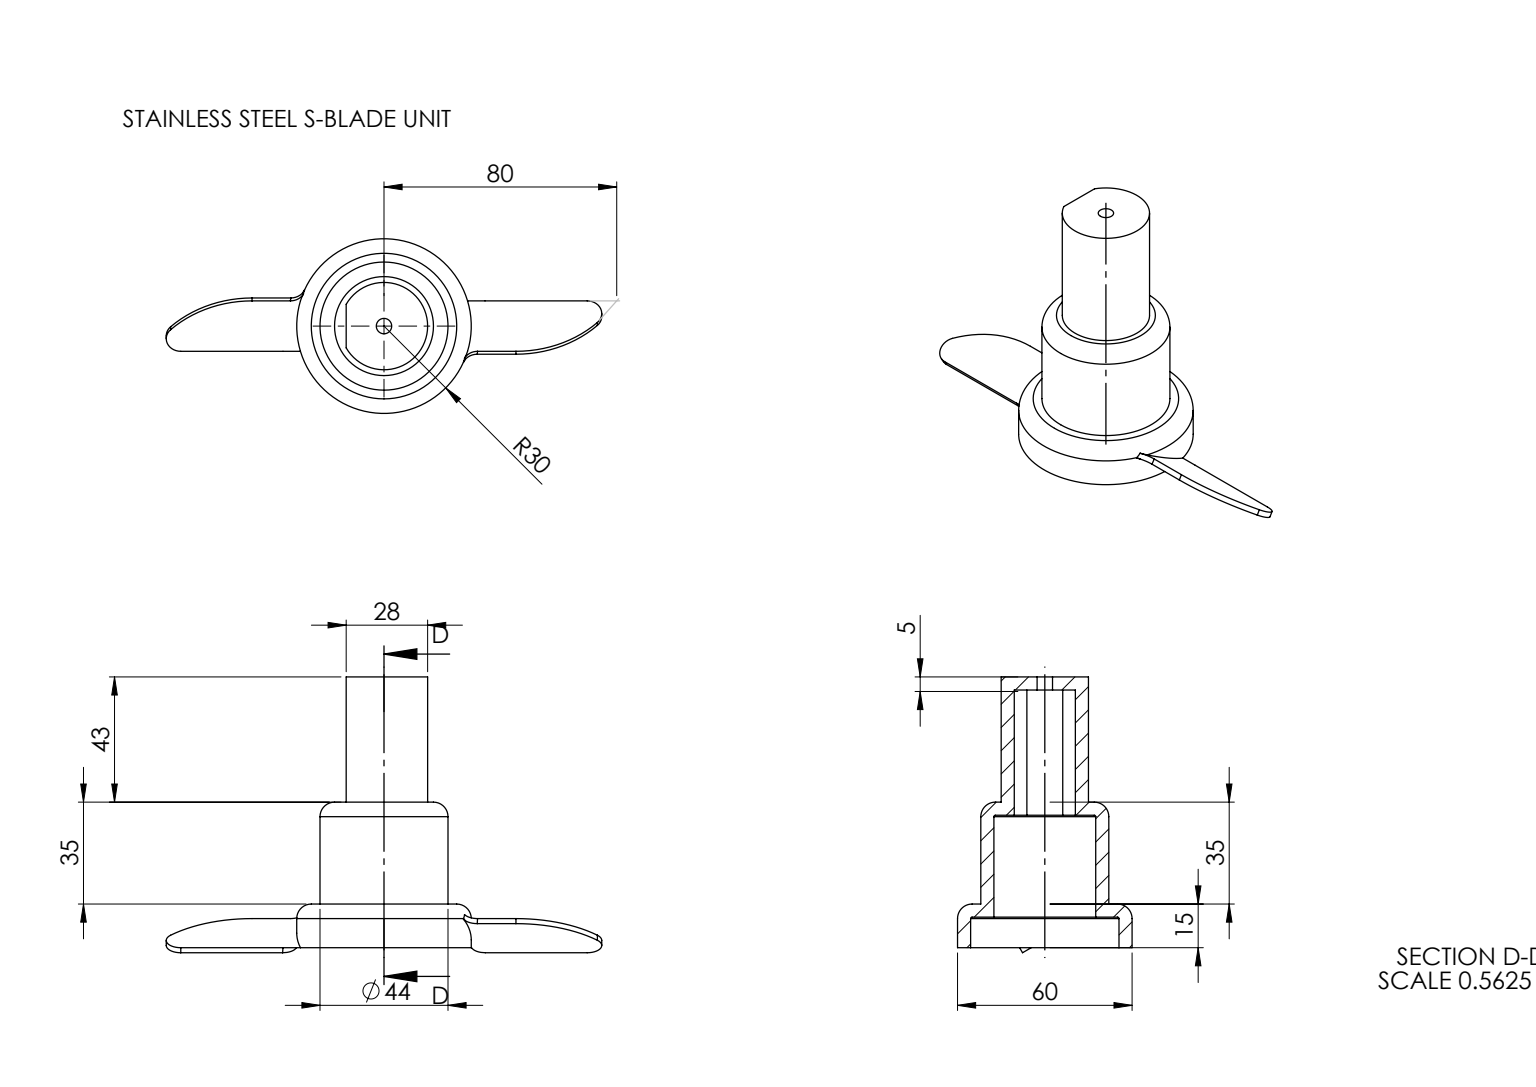
ISO-10303-21;
HEADER;
FILE_DESCRIPTION (('STEP AP214'),
    '1' );
FILE_NAME ('Stainless Steel S-Blade Unit.step',
    '2026-10-08T14:59:03',
    ( '' ),
    ( '' ),
    'SwSTEP 2.0',
    'SolidWorks 2026',
    '' );
FILE_SCHEMA (( 'AUTOMOTIVE_DESIGN' ));
ENDSEC;

DATA;
#5=LINE ( 'NONE', #4817, #10432 ) ;
#8=VERTEX_POINT ( 'NONE', #10428 ) ;
#24=DIRECTION ( 'NONE',  ( 0.000000000000000000, 0.000000000000000000, -1.000000000000000000 ) ) ;
#25=CARTESIAN_POINT ( 'NONE',  ( -30.63265341208206038, 76.40790137508867019, 5.685798939282528330 ) ) ;
#48=EDGE_LOOP ( 'NONE', ( #1031, #6053, #2883, #3031 ) ) ;
#49=CARTESIAN_POINT ( 'NONE',  ( 30.43737458073258040, 77.00000000000001421, -5.702507482421638407 ) ) ;
#59=DIRECTION ( 'NONE',  ( 0.000000000000000000, -0.4999999999999976685, 0.8660254037844399289 ) ) ;
#68=AXIS2_PLACEMENT_3D ( 'NONE', #1472, #532, #4327 ) ;
#76=ORIENTED_EDGE ( 'NONE', *, *, #6927, .T. ) ;
#80=VERTEX_POINT ( 'NONE', #3761 ) ;
#106=DIRECTION ( 'NONE',  ( -0.000000000000000000, -1.000000000000000000, -0.000000000000000000 ) ) ;
#111=ORIENTED_EDGE ( 'NONE', *, *, #6676, .F. ) ;
#114=CARTESIAN_POINT ( 'NONE',  ( 27.33018067101281900, 86.99999999999998579, 12.37179148263487782 ) ) ;
#142=EDGE_LOOP ( 'NONE', ( #5615, #3837, #7263, #6163, #8146, #5499, #6846 ) ) ;
#144=DIRECTION ( 'NONE',  ( -0.000000000000000000, -1.000000000000000000, -0.000000000000000000 ) ) ;
#151=ORIENTED_EDGE ( 'NONE', *, *, #4389, .T. ) ;
#174=CARTESIAN_POINT ( 'NONE',  ( 30.14540500433760783, 76.99999999999997158, -4.927060346216586950 ) ) ;
#181=DIRECTION ( 'NONE',  ( 0.000000000000000000, -0.000000000000000000, 1.000000000000000000 ) ) ;
#182=ORIENTED_EDGE ( 'NONE', *, *, #8491, .F. ) ;
#188=LINE ( 'NONE', #3126, #12048 ) ;
#189=ORIENTED_EDGE ( 'NONE', *, *, #4744, .F. ) ;
#205=ORIENTED_EDGE ( 'NONE', *, *, #4032, .F. ) ;
#207=PRODUCT ( 'Stainless Steel S-Blade Unit', 'Stainless Steel S-Blade Unit', '', ( #412 ) ) ;
#221=TOROIDAL_SURFACE ( 'NONE', #8577, 17.00000000000000000, 5.000000000000000000 ) ;
#224=ADVANCED_FACE ( 'NONE', ( #10291 ), #7552, .F. ) ;
#226=CARTESIAN_POINT ( 'NONE',  ( 31.26438337082144159, 85.29075299833057500, 9.699751388268191832 ) ) ;
#227=CARTESIAN_POINT ( 'NONE',  ( 3.245314017740478073E-16, 170.0000000000000000, -2.649999999999993694 ) ) ;
#228=FACE_OUTER_BOUND ( 'NONE', #12039, .T. ) ;
#230=EDGE_LOOP ( 'NONE', ( #6810, #2498, #7329, #11688 ) ) ;
#247=CYLINDRICAL_SURFACE ( 'NONE', #2591, 40.00000000000000000 ) ;
#248=EDGE_CURVE ( 'NONE', #3797, #2264, #8566, .T. ) ;
#268=ORIENTED_EDGE ( 'NONE', *, *, #4405, .T. ) ;
#281=EDGE_LOOP ( 'NONE', ( #4160, #1583, #966, #3668, #2740 ) ) ;
#283=DIRECTION ( 'NONE',  ( 1.224646799147352714E-16, 0.000000000000000000, -1.000000000000000000 ) ) ;
#293=ADVANCED_FACE ( 'NONE', ( #5930 ), #247, .T. ) ;
#302=VECTOR ( 'NONE', #2224, 1000.000000000000000 ) ;
#311=AXIS2_PLACEMENT_3D ( 'NONE', #7560, #9353, #11370 ) ;
#330=B_SPLINE_CURVE_WITH_KNOTS ( 'NONE', 3,
 ( #6794, #1186, #6609, #4798, #1865, #11603, #5861, #4988, #8525, #7602, #9644, #2863, #10471, #8586, #49, #3865, #174, #7662 ),
 .UNSPECIFIED., .F., .F.,
 ( 4, 2, 2, 2, 2, 2, 2, 2, 4 ),
 ( 2.823925224926892107E-17, 0.0008221565609605404907, 0.001644313121921052792, 0.002466469682881565310, 0.003288626243842077395, 0.004110782804802590347, 0.004932939365763108937, 0.005755095926723627527, 0.006577252487684147851 ),
 .UNSPECIFIED. ) ;
#331=ORIENTED_EDGE ( 'NONE', *, *, #3823, .F. ) ;
#334=VERTEX_POINT ( 'NONE', #4888 ) ;
#373=CARTESIAN_POINT ( 'NONE',  ( 0.000000000000000000, 87.00000000000000000, 0.000000000000000000 ) ) ;
#380=DIRECTION ( 'NONE',  ( 1.000000000000000000, 0.000000000000000000, 0.000000000000000000 ) ) ;
#386=( GEOMETRIC_REPRESENTATION_CONTEXT ( 3 ) GLOBAL_UNCERTAINTY_ASSIGNED_CONTEXT ( ( #5659 ) ) GLOBAL_UNIT_ASSIGNED_CONTEXT ( ( #9241, #4519, #9302 ) ) REPRESENTATION_CONTEXT ( 'NONE', 'WORKASPACE' ) );
#396=CIRCLE ( 'NONE', #7375, 0.5000000000000004441 ) ;
#397=APPLICATION_CONTEXT ( 'automotive_design' ) ;
#408=EDGE_CURVE ( 'NONE', #10035, #8931, #706, .T. ) ;
#412=PRODUCT_CONTEXT ( 'NONE', #6769, 'mechanical' ) ;
#420=TOROIDAL_SURFACE ( 'NONE', #1423, 17.00000000000000000, 5.000000000000000000 ) ;
#422=CARTESIAN_POINT ( 'NONE',  ( 27.33018067101282966, 87.00000000000000000, 12.37179148263486539 ) ) ;
#425=CARTESIAN_POINT ( 'NONE',  ( 1.285879139104720633E-15, 216.0365690573663926, 10.49999999999999822 ) ) ;
#426=EDGE_LOOP ( 'NONE', ( #189, #2218, #6237, #8413 ) ) ;
#427=CIRCLE ( 'NONE', #3428, 30.00000000000000000 ) ;
#429=AXIS2_PLACEMENT_3D ( 'NONE', #2506, #6308, #1510 ) ;
#430=CARTESIAN_POINT ( 'NONE',  ( -30.34950626935404827, 87.16600977219412982, -8.947791397837656646 ) ) ;
#432=DIRECTION ( 'NONE',  ( 0.000000000000000000, 0.000000000000000000, 1.000000000000000000 ) ) ;
#446=LINE ( 'NONE', #10918, #2988 ) ;
#459=DIRECTION ( 'NONE',  ( 0.000000000000000000, 0.000000000000000000, 1.000000000000000000 ) ) ;
#471=CARTESIAN_POINT ( 'NONE',  ( 30.49437064397536901, 76.52118294276679933, -5.489589508502957571 ) ) ;
#497=ORIENTED_EDGE ( 'NONE', *, *, #5720, .F. ) ;
#498=DIRECTION ( 'NONE',  ( -0.000000000000000000, -1.000000000000000000, -0.000000000000000000 ) ) ;
#506=CARTESIAN_POINT ( 'NONE',  ( -29.63582346253862454, 77.00000000000000000, 4.660254037844413944 ) ) ;
#532=DIRECTION ( 'NONE',  ( 0.000000000000000000, 1.000000000000000000, 0.000000000000000000 ) ) ;
#534=CARTESIAN_POINT ( 'NONE',  ( 27.30107202361637775, 86.87046582918780757, 12.43589427268144831 ) ) ;
#535=CARTESIAN_POINT ( 'NONE',  ( 30.15809951803416666, 76.87504465863048608, -4.876683037773544172 ) ) ;
#536=CARTESIAN_POINT ( 'NONE',  ( 0.000000000000000000, 170.0000000000000000, 0.000000000000000000 ) ) ;
#545=PRODUCT_DEFINITION ( 'UNKNOWN', '', #11724, #3142 ) ;
#556=CIRCLE ( 'NONE', #11914, 10.49999999999999822 ) ;
#570=FACE_OUTER_BOUND ( 'NONE', #48, .T. ) ;
#579=DIRECTION ( 'NONE',  ( -1.000000000000000000, 0.000000000000000000, 0.000000000000000000 ) ) ;
#593=DIRECTION ( 'NONE',  ( 0.000000000000000000, 1.000000000000000000, 0.000000000000000000 ) ) ;
#601=CARTESIAN_POINT ( 'NONE',  ( -27.65415084186107109, 87.92311536631548563, -11.47631757750353643 ) ) ;
#614=CARTESIAN_POINT ( 'NONE',  ( 27.65415084186298245, 87.92311536631358138, 11.47631757750026438 ) ) ;
#620=CARTESIAN_POINT ( 'NONE',  ( -27.67899820261485999, 88.38261385519929547, -11.05501148229834030 ) ) ;
#621=ORIENTED_EDGE ( 'NONE', *, *, #3640, .F. ) ;
#625=CIRCLE ( 'NONE', #4207, 5.000000000000000888 ) ;
#626=CARTESIAN_POINT ( 'NONE',  ( 31.12930703771215235, 75.68563247576862807, -7.901403593909491541 ) ) ;
#630=CARTESIAN_POINT ( 'NONE',  ( 69.85388127645428824, 79.49999999999998579, -4.330127018922231841 ) ) ;
#635=CYLINDRICAL_SURFACE ( 'NONE', #1812, 30.00000000000000000 ) ;
#638=EDGE_CURVE ( 'NONE', #7703, #7018, #7140, .T. ) ;
#640=CARTESIAN_POINT ( 'NONE',  ( 27.65180490099799115, 87.90152798314358051, 11.49631016393330540 ) ) ;
#647=ORIENTED_EDGE ( 'NONE', *, *, #8392, .F. ) ;
#657=FILL_AREA_STYLE_COLOUR ( '', #970 ) ;
#661=CARTESIAN_POINT ( 'NONE',  ( -45.35898384862240107, 86.99999999999997158, -8.660254037844424602 ) ) ;
#670=CYLINDRICAL_SURFACE ( 'NONE', #2203, 10.49999999999999822 ) ;
#671=EDGE_CURVE ( 'NONE', #7769, #10587, #7043, .T. ) ;
#674=CYLINDRICAL_SURFACE ( 'NONE', #5648, 15.00000000000000000 ) ;
#676=CARTESIAN_POINT ( 'NONE',  ( -30.00100000000000122, 77.00000000000000000, -8.660254037844445918 ) ) ;
#683=ADVANCED_FACE ( 'NONE', ( #4455, #3529 ), #8312, .T. ) ;
#688=CARTESIAN_POINT ( 'NONE',  ( 34.77127485704751564, 76.44489695195846934, -8.339765143629700006 ) ) ;
#691=DIRECTION ( 'NONE',  ( 0.000000000000000000, -0.8660254037844407060, -0.4999999999999965028 ) ) ;
#696=CYLINDRICAL_SURFACE ( 'NONE', #1896, 17.50000000000000000 ) ;
#703=DIRECTION ( 'NONE',  ( 1.000000000000000000, 0.000000000000000000, 0.000000000000000000 ) ) ;
#706=B_SPLINE_CURVE_WITH_KNOTS ( 'NONE', 3,
 ( #3890, #11502, #7747, #11561 ),
 .UNSPECIFIED., .F., .F.,
 ( 4, 4 ),
 ( 0.000000000000000000, 0.001357209897699670955 ),
 .UNSPECIFIED. ) ;
#718=FACE_OUTER_BOUND ( 'NONE', #11904, .T. ) ;
#721=DIRECTION ( 'NONE',  ( -0.000000000000000000, -1.000000000000000000, -0.000000000000000000 ) ) ;
#722=CIRCLE ( 'NONE', #921, 40.00000000000000000 ) ;
#724=EDGE_LOOP ( 'NONE', ( #7478, #11917, #621, #1398 ) ) ;
#726=B_SPLINE_CURVE_WITH_KNOTS ( 'NONE', 3,
 ( #5759, #4688, #1765, #8421 ),
 .UNSPECIFIED., .F., .F.,
 ( 4, 4 ),
 ( 0.000000000000000000, 0.002001274951694169153 ),
 .UNSPECIFIED. ) ;
#734=CARTESIAN_POINT ( 'NONE',  ( 0.000000000000000000, 127.0000000000000000, 0.000000000000000000 ) ) ;
#742=EDGE_LOOP ( 'NONE', ( #9342, #3526, #10485, #11102, #11036 ) ) ;
#747=ADVANCED_FACE ( 'NONE', ( #10001, #3466 ), #7268, .F. ) ;
#748=DIRECTION ( 'NONE',  ( 0.000000000000000000, 0.000000000000000000, 1.000000000000000000 ) ) ;
#751=ORIENTED_EDGE ( 'NONE', *, *, #7330, .F. ) ;
#754=DIRECTION ( 'NONE',  ( 0.000000000000000000, 1.000000000000000000, 0.000000000000000000 ) ) ;
#757=ORIENTED_EDGE ( 'NONE', *, *, #11505, .F. ) ;
#759=CARTESIAN_POINT ( 'NONE',  ( -34.72842983617974966, 77.03714026276665550, 8.681696978550554888 ) ) ;
#763=MANIFOLD_SOLID_BREP ( 'M5 Clearance Hole1', #5696 ) ;
#771=CARTESIAN_POINT ( 'NONE',  ( 27.52813290908668264, 87.44182241851449078, 11.93450069589769136 ) ) ;
#773=AXIS2_PLACEMENT_3D ( 'NONE', #816, #4609, #12225 ) ;
#781=CARTESIAN_POINT ( 'NONE',  ( -45.35898384862240107, 65.26794919243121740, 24.98076211353317078 ) ) ;
#784=DIRECTION ( 'NONE',  ( 0.000000000000000000, 0.000000000000000000, -1.000000000000000000 ) ) ;
#802=ORIENTED_EDGE ( 'NONE', *, *, #6455, .F. ) ;
#807=CIRCLE ( 'NONE', #9945, 5.000000000000000888 ) ;
#813=AXIS2_PLACEMENT_3D ( 'NONE', #4855, #106, #2049 ) ;
#816=CARTESIAN_POINT ( 'NONE',  ( 0.000000000000000000, 122.5000000000000000, 0.000000000000000000 ) ) ;
#817=DIRECTION ( 'NONE',  ( 0.000000000000000000, 0.000000000000000000, 1.000000000000000000 ) ) ;
#820=CARTESIAN_POINT ( 'NONE',  ( -31.06657576416735012, 76.26187158480907158, 8.234095398640720376 ) ) ;
#852=CARTESIAN_POINT ( 'NONE',  ( -31.33267436902169933, 77.00000000000000000, 7.087639215986555108 ) ) ;
#864=CARTESIAN_POINT ( 'NONE',  ( 0.000000000000000000, 127.0000000000000000, 0.000000000000000000 ) ) ;
#870=CARTESIAN_POINT ( 'NONE',  ( 0.000000000000000000, 77.00000000000000000, 0.000000000000000000 ) ) ;
#897=EDGE_CURVE ( 'NONE', #5507, #7525, #3143, .T. ) ;
#898=ORIENTED_EDGE ( 'NONE', *, *, #2970, .F. ) ;
#913=DIRECTION ( 'NONE',  ( -0.000000000000000000, -1.000000000000000000, -0.000000000000000000 ) ) ;
#921=AXIS2_PLACEMENT_3D ( 'NONE', #781, #3754, #11121 ) ;
#922=UNCERTAINTY_MEASURE_WITH_UNIT (LENGTH_MEASURE( 1.000000000000000082E-05 ), #12072, 'distance_accuracy_value', 'NONE');
#928=CARTESIAN_POINT ( 'NONE',  ( 0.000000000000000000, 170.0000000000000000, 2.649999999999987477 ) ) ;
#929=DIRECTION ( 'NONE',  ( -0.000000000000000000, -1.000000000000000000, -0.000000000000000000 ) ) ;
#931=VERTEX_POINT ( 'NONE', #10744 ) ;
#941=ORIENTED_EDGE ( 'NONE', *, *, #1209, .F. ) ;
#944=DIRECTION ( 'NONE',  ( 0.000000000000000000, 0.000000000000000000, 1.000000000000000000 ) ) ;
#945=VERTEX_POINT ( 'NONE', #2266 ) ;
#948=CYLINDRICAL_SURFACE ( 'NONE', #5812, 25.50000000000000000 ) ;
#949=CARTESIAN_POINT ( 'NONE',  ( 0.000000000000000000, 122.0000000000000000, 0.000000000000000000 ) ) ;
#954=ORIENTED_EDGE ( 'NONE', *, *, #1330, .T. ) ;
#955=FACE_OUTER_BOUND ( 'NONE', #3507, .T. ) ;
#957=DIRECTION ( 'NONE',  ( 1.000000000000000000, 0.000000000000000000, 0.000000000000000000 ) ) ;
#966=ORIENTED_EDGE ( 'NONE', *, *, #9420, .T. ) ;
#970=COLOUR_RGB ( '', 0.72549020, 0.75294118, 0.79215686) ;
#973=EDGE_CURVE ( 'NONE', #8579, #2134, #1216, .T. ) ;
#993=ORIENTED_EDGE ( 'NONE', *, *, #10766, .F. ) ;
#998=ORIENTED_EDGE ( 'NONE', *, *, #9593, .T. ) ;
#1003=CARTESIAN_POINT ( 'NONE',  ( 73.35315233757310693, 81.28571428571424917, -1.237179148263527928 ) ) ;
#1009=ORIENTED_EDGE ( 'NONE', *, *, #2846, .T. ) ;
#1031=ORIENTED_EDGE ( 'NONE', *, *, #1499, .F. ) ;
#1044=DIRECTION ( 'NONE',  ( 0.000000000000000000, 0.000000000000000000, 1.000000000000000000 ) ) ;
#1045=CARTESIAN_POINT ( 'NONE',  ( -30.00100000000000122, 87.00000000000000000, 8.660254037844435260 ) ) ;
#1049=DIRECTION ( 'NONE',  ( 0.000000000000000000, 0.000000000000000000, 1.000000000000000000 ) ) ;
#1058=EDGE_LOOP ( 'NONE', ( #182, #7997, #8845 ) ) ;
#1069=AXIS2_PLACEMENT_3D ( 'NONE', #1304, #9952, #1425 ) ;
#1071=EDGE_CURVE ( 'NONE', #4547, #3216, #10105, .T. ) ;
#1084=DIRECTION ( 'NONE',  ( -1.000000000000000000, 0.000000000000000000, 0.000000000000000000 ) ) ;
#1086=FACE_OUTER_BOUND ( 'NONE', #6691, .T. ) ;
#1091=CIRCLE ( 'NONE', #12038, 2.649999999999993694 ) ;
#1106=AXIS2_PLACEMENT_3D ( 'NONE', #9506, #3916, #8635 ) ;
#1108=CARTESIAN_POINT ( 'NONE',  ( 32.05000697088088657, 85.26794919243110371, 9.660254037844429931 ) ) ;
#1109=CARTESIAN_POINT ( 'NONE',  ( 0.000000000000000000, 170.0000000000000000, 0.000000000000000000 ) ) ;
#1112=VERTEX_POINT ( 'NONE', #10048 ) ;
#1155=DIRECTION ( 'NONE',  ( 0.000000000000000000, 0.000000000000000000, 1.000000000000000000 ) ) ;
#1159=CARTESIAN_POINT ( 'NONE',  ( -31.48070082314331231, 75.91043305631261262, 6.547439342558601716 ) ) ;
#1169=( BOUNDED_CURVE ( )  B_SPLINE_CURVE ( 3, ( #7961, #10837, #3366, #8897 ),
 .UNSPECIFIED., .F., .F. ) 
 B_SPLINE_CURVE_WITH_KNOTS ( ( 4, 4 ),
 ( 1.143370257677567281, 1.145717000886475878 ),
 .UNSPECIFIED. ) 
 CURVE ( )  GEOMETRIC_REPRESENTATION_ITEM ( )  RATIONAL_B_SPLINE_CURVE ( ( 1.000000000000000000, 0.9999995410664119788, 0.9999995410664119788, 1.000000000000000000 ) ) 
 REPRESENTATION_ITEM ( '' )  );
#1177=EDGE_CURVE ( 'NONE', #334, #8, #726, .T. ) ;
#1183=CARTESIAN_POINT ( 'NONE',  ( -69.85388127645425982, 75.26794919243111792, 7.660254037844449471 ) ) ;
#1186=CARTESIAN_POINT ( 'NONE',  ( 34.45294269781049223, 77.00000000000002842, -8.660253777987195534 ) ) ;
#1203=PLANE ( 'NONE',  #10847 ) ;
#1208=CARTESIAN_POINT ( 'NONE',  ( -73.35315233757310693, 79.55366347814538130, 0.2371791482635408899 ) ) ;
#1209=EDGE_CURVE ( 'NONE', #931, #7101, #5, .T. ) ;
#1216=LINE ( 'NONE', #10621, #3070 ) ;
#1230=DIRECTION ( 'NONE',  ( -0.000000000000000000, 1.000000000000000000, -0.000000000000000000 ) ) ;
#1246=CARTESIAN_POINT ( 'NONE',  ( 27.32044479829590244, 86.95653975047672191, 12.39329872843003066 ) ) ;
#1255=ORIENTED_EDGE ( 'NONE', *, *, #4032, .T. ) ;
#1257=CARTESIAN_POINT ( 'NONE',  ( 29.92433840049366012, 87.25972750007186107, 9.110115264091716014 ) ) ;
#1273=VECTOR ( 'NONE', #6369, 1000.000000000000000 ) ;
#1284=VECTOR ( 'NONE', #579, 1000.000000000000000 ) ;
#1285=AXIS2_PLACEMENT_3D ( 'NONE', #870, #2729, #748 ) ;
#1293=CARTESIAN_POINT ( 'NONE',  ( -45.35898384862240107, 67.00000000000008527, 25.98076211353315657 ) ) ;
#1294=CARTESIAN_POINT ( 'NONE',  ( -28.72281323269012532, 77.00000000000000000, 8.660254037844445918 ) ) ;
#1298=VECTOR ( 'NONE', #12093, 1000.000000000000000 ) ;
#1301=EDGE_CURVE ( 'NONE', #5989, #7101, #10232, .T. ) ;
#1304=CARTESIAN_POINT ( 'NONE',  ( 0.000000000000000000, 87.50000000000000000, 0.000000000000000000 ) ) ;
#1307=CARTESIAN_POINT ( 'NONE',  ( 30.00100000000000122, 77.00000000000000000, 8.660254037844445918 ) ) ;
#1309=VECTOR ( 'NONE', #6876, 1000.000000000000000 ) ;
#1318=DIRECTION ( 'NONE',  ( 0.000000000000000000, 0.000000000000000000, 1.000000000000000000 ) ) ;
#1330=EDGE_CURVE ( 'NONE', #7513, #6899, #8632, .T. ) ;
#1364=CARTESIAN_POINT ( 'NONE',  ( 34.73110591274434000, 77.00000000000000000, -8.660254037844445918 ) ) ;
#1368=CARTESIAN_POINT ( 'NONE',  ( -29.32777202433393526, 87.43477800909944619, -9.413311639618301641 ) ) ;
#1386=CARTESIAN_POINT ( 'NONE',  ( 28.72281323269012532, 87.00000000000000000, 8.660254037844435260 ) ) ;
#1393=ORIENTED_EDGE ( 'NONE', *, *, #5864, .F. ) ;
#1398=ORIENTED_EDGE ( 'NONE', *, *, #4341, .T. ) ;
#1399=CARTESIAN_POINT ( 'NONE',  ( 45.35898384862240107, 5.499999999999840128, 9.526279441628638267 ) ) ;
#1409=AXIS2_PLACEMENT_3D ( 'NONE', #11572, #5209, #459 ) ;
#1413=CARTESIAN_POINT ( 'NONE',  ( 30.00100000000000122, 87.00000000000000000, -8.660254037844435260 ) ) ;
#1414=CIRCLE ( 'NONE', #5603, 22.00000000000000355 ) ;
#1415=CARTESIAN_POINT ( 'NONE',  ( 33.79339916392899568, 75.30908861350523864, -7.588998470350058589 ) ) ;
#1423=AXIS2_PLACEMENT_3D ( 'NONE', #949, #4556, #8530 ) ;
#1425=DIRECTION ( 'NONE',  ( 0.000000000000000000, 0.000000000000000000, 1.000000000000000000 ) ) ;
#1426=ORIENTED_EDGE ( 'NONE', *, *, #1301, .F. ) ;
#1436=ORIENTED_EDGE ( 'NONE', *, *, #4623, .T. ) ;
#1439=LINE ( 'NONE', #11859, #12313 ) ;
#1443=CARTESIAN_POINT ( 'NONE',  ( 0.000000000000000000, 127.0000000000000000, 0.000000000000000000 ) ) ;
#1445=ORIENTED_EDGE ( 'NONE', *, *, #1071, .F. ) ;
#1448=CARTESIAN_POINT ( 'NONE',  ( -30.55518048406710818, 80.37544454677752981, -1.186187415305626436 ) ) ;
#1449=DIRECTION ( 'NONE',  ( 0.000000000000000000, 0.000000000000000000, -1.000000000000000000 ) ) ;
#1450=ORIENTED_EDGE ( 'NONE', *, *, #3823, .T. ) ;
#1453=ORIENTED_EDGE ( 'NONE', *, *, #9437, .F. ) ;
#1454=EDGE_CURVE ( 'NONE', #7484, #7525, #4811, .T. ) ;
#1472=CARTESIAN_POINT ( 'NONE',  ( 0.000000000000000000, 77.00000000000000000, 0.000000000000000000 ) ) ;
#1482=CARTESIAN_POINT ( 'NONE',  ( 69.85388127645425982, 75.26794919243111792, -7.660254037844449471 ) ) ;
#1486=CARTESIAN_POINT ( 'NONE',  ( 31.88521078284829713, 87.00000000000001421, 14.43375672974067569 ) ) ;
#1499=EDGE_CURVE ( 'NONE', #9385, #11869, #4012, .T. ) ;
#1510=DIRECTION ( 'NONE',  ( 0.000000000000000000, -0.4999999999999976130, -0.8660254037844400399 ) ) ;
#1513=CARTESIAN_POINT ( 'NONE',  ( 28.47250777504872588, 87.47929846073044757, 9.490423323819145551 ) ) ;
#1538=CARTESIAN_POINT ( 'NONE',  ( -31.92904760676809062, 76.99999999999998579, 7.658217335466646070 ) ) ;
#1548=ORIENTED_EDGE ( 'NONE', *, *, #4290, .T. ) ;
#1554=DIRECTION ( 'NONE',  ( 0.000000000000000000, 1.000000000000000000, 0.000000000000000000 ) ) ;
#1557=CARTESIAN_POINT ( 'NONE',  ( -28.14852131675075242, 87.98519278820045031, -10.36665800225805967 ) ) ;
#1558=ADVANCED_FACE ( 'NONE', ( #11038 ), #221, .T. ) ;
#1559=ORIENTED_EDGE ( 'NONE', *, *, #6927, .F. ) ;
#1569=VERTEX_POINT ( 'NONE', #3245 ) ;
#1583=ORIENTED_EDGE ( 'NONE', *, *, #4955, .T. ) ;
#1593=DIRECTION ( 'NONE',  ( 0.000000000000000000, 1.000000000000000000, 0.000000000000000000 ) ) ;
#1600=CARTESIAN_POINT ( 'NONE',  ( -27.56105762898379652, 86.58728811733517716, -11.86287969473305814 ) ) ;
#1607=ADVANCED_FACE ( 'NONE', ( #4426 ), #8219, .F. ) ;
#1612=AXIS2_PLACEMENT_3D ( 'NONE', #9562, #7823, #5032 ) ;
#1614=DIRECTION ( 'NONE',  ( 0.000000000000000000, 0.8660254037844405950, 0.4999999999999965028 ) ) ;
#1617=CARTESIAN_POINT ( 'NONE',  ( 27.96741528345890870, 86.27927944434865992, 11.41192941739706335 ) ) ;
#1626=CARTESIAN_POINT ( 'NONE',  ( 2.081899558550500280E-15, 122.0000000000000000, -17.00000000000000000 ) ) ;
#1630=AXIS2_PLACEMENT_3D ( 'NONE', #2809, #11358, #8265 ) ;
#1637=DIRECTION ( 'NONE',  ( 1.224646799147357151E-16, 0.000000000000000000, -1.000000000000000000 ) ) ;
#1642=DIRECTION ( 'NONE',  ( -0.000000000000000000, -1.000000000000000000, -0.000000000000000000 ) ) ;
#1643=( BOUNDED_CURVE ( )  B_SPLINE_CURVE ( 3, ( #3135, #10732, #5077, #8852 ),
 .UNSPECIFIED., .F., .F. ) 
 B_SPLINE_CURVE_WITH_KNOTS ( ( 4, 4 ),
 ( 1.666086958916892291, 1.694832046014206117 ),
 .UNSPECIFIED. ) 
 CURVE ( )  GEOMETRIC_REPRESENTATION_ITEM ( )  RATIONAL_B_SPLINE_CURVE ( ( 1.000000000000000000, 0.9999311445159493328, 0.9999311445159493328, 1.000000000000000000 ) ) 
 REPRESENTATION_ITEM ( '' )  );
#1653=ORIENTED_EDGE ( 'NONE', *, *, #8115, .F. ) ;
#1657=EDGE_CURVE ( 'NONE', #3216, #11487, #625, .T. ) ;
#1659=CARTESIAN_POINT ( 'NONE',  ( -34.45294269781049223, 77.00000000000002842, 8.660253777987195534 ) ) ;
#1661=CARTESIAN_POINT ( 'NONE',  ( -28.82113438504157799, 85.77482169909444565, -9.367611059671812512 ) ) ;
#1663=CARTESIAN_POINT ( 'NONE',  ( 1.285879139104720633E-15, 165.5000000000000000, 10.49999999999999822 ) ) ;
#1667=ADVANCED_FACE ( 'NONE', ( #3848 ), #10176, .T. ) ;
#1671=STYLED_ITEM ( 'NONE', ( #11321 ), #763 ) ;
#1675=CARTESIAN_POINT ( 'NONE',  ( -69.85388127645428824, 75.26794919243114634, 7.660254037844465458 ) ) ;
#1677=DIRECTION ( 'NONE',  ( -0.000000000000000000, -1.000000000000000000, -0.000000000000000000 ) ) ;
#1679=EDGE_LOOP ( 'NONE', ( #3569, #5275 ) ) ;
#1685=CARTESIAN_POINT ( 'NONE',  ( 31.18707241436460365, 75.10640101998821194, -7.566984156997462740 ) ) ;
#1689=DIRECTION ( 'NONE',  ( 0.000000000000000000, 1.000000000000000000, 0.000000000000000000 ) ) ;
#1690=CARTESIAN_POINT ( 'NONE',  ( -34.84179752789421514, 75.25738092153642356, 7.654152443798540872 ) ) ;
#1705=PLANE ( 'NONE',  #7184 ) ;
#1718=SURFACE_STYLE_USAGE ( .BOTH. , #10116 ) ;
#1719=AXIS2_PLACEMENT_3D ( 'NONE', #8085, #1554, #2298 ) ;
#1720=CIRCLE ( 'NONE', #8675, 5.000000000000000000 ) ;
#1723=CARTESIAN_POINT ( 'NONE',  ( -30.55702146375036676, 77.00000000000001421, 5.949569453687718834 ) ) ;
#1732=AXIS2_PLACEMENT_3D ( 'NONE', #4755, #7623, #8611 ) ;
#1736=DIRECTION ( 'NONE',  ( 0.000000000000000000, 0.000000000000000000, 1.000000000000000000 ) ) ;
#1739=FACE_BOUND ( 'NONE', #6832, .T. ) ;
#1745=CARTESIAN_POINT ( 'NONE',  ( 31.06657576416735012, 76.26187158480907158, -8.234095398640720376 ) ) ;
#1746=CARTESIAN_POINT ( 'NONE',  ( 30.43816488677641630, 83.71535165408627677, 2.971076217724753832 ) ) ;
#1756=CIRCLE ( 'NONE', #10100, 10.49999999999999822 ) ;
#1760=EDGE_CURVE ( 'NONE', #5507, #8953, #9981, .T. ) ;
#1761=ORIENTED_EDGE ( 'NONE', *, *, #7465, .F. ) ;
#1765=CARTESIAN_POINT ( 'NONE',  ( 32.14616437604218646, 85.84037417286381810, 9.329764321300741514 ) ) ;
#1778=CARTESIAN_POINT ( 'NONE',  ( -30.83210227225915290, 77.00000000000000000, 6.426308247889123137 ) ) ;
#1783=LINE ( 'NONE', #9186, #2910 ) ;
#1793=VERTEX_POINT ( 'NONE', #8756 ) ;
#1795=DIRECTION ( 'NONE',  ( 0.000000000000000000, 0.000000000000000000, 1.000000000000000000 ) ) ;
#1799=B_SPLINE_CURVE_WITH_KNOTS ( 'NONE', 3,
 ( #9122, #535, #10819, #471, #4398, #9817, #7147, #7089, #3412, #11832, #10944, #1415, #12015, #8193 ),
 .UNSPECIFIED., .F., .F.,
 ( 4, 2, 2, 2, 2, 2, 4 ),
 ( 0.001978049138782353184, 0.002761379211137155940, 0.003544709283491958261, 0.004328039355846760583, 0.005111369428201563772, 0.006678029572911168416, 0.008244689717620771324 ),
 .UNSPECIFIED. ) ;
#1812=AXIS2_PLACEMENT_3D ( 'NONE', #4187, #3447, #1449 ) ;
#1822=EDGE_CURVE ( 'NONE', #9024, #5307, #10195, .T. ) ;
#1825=ORIENTED_EDGE ( 'NONE', *, *, #7480, .T. ) ;
#1827=CYLINDRICAL_SURFACE ( 'NONE', #311, 10.49999999999999822 ) ;
#1828=ORIENTED_EDGE ( 'NONE', *, *, #2846, .F. ) ;
#1831=AXIS2_PLACEMENT_3D ( 'NONE', #10884, #3158, #9815 ) ;
#1834=VERTEX_POINT ( 'NONE', #6029 ) ;
#1836=EDGE_CURVE ( 'NONE', #10799, #1569, #9879, .T. ) ;
#1837=CARTESIAN_POINT ( 'NONE',  ( 0.000000000000000000, 92.00000000000000000, -25.50000000000000000 ) ) ;
#1840=DIRECTION ( 'NONE',  ( -1.000000000000000000, 0.000000000000000000, 0.000000000000000000 ) ) ;
#1845=EDGE_CURVE ( 'NONE', #1793, #9034, #5023, .T. ) ;
#1854=AXIS2_PLACEMENT_3D ( 'NONE', #4718, #10633, #4846 ) ;
#1858=ORIENTED_EDGE ( 'NONE', *, *, #1499, .T. ) ;
#1865=CARTESIAN_POINT ( 'NONE',  ( 33.37417589188917333, 76.99999999999998579, -8.451338748825380165 ) ) ;
#1872=VECTOR ( 'NONE', #9243, 1000.000000000000000 ) ;
#1873=ORIENTED_EDGE ( 'NONE', *, *, #897, .F. ) ;
#1879=FACE_BOUND ( 'NONE', #2862, .T. ) ;
#1881=ORIENTED_EDGE ( 'NONE', *, *, #6930, .T. ) ;
#1882=VECTOR ( 'NONE', #957, 1000.000000000000000 ) ;
#1885=EDGE_LOOP ( 'NONE', ( #8424, #7096, #8090, #5651 ) ) ;
#1886=EDGE_CURVE ( 'NONE', #2508, #11122, #427, .T. ) ;
#1896=AXIS2_PLACEMENT_3D ( 'NONE', #10342, #2625, #9283 ) ;
#1897=EDGE_LOOP ( 'NONE', ( #10651, #7896, #3999, #10787, #1426, #9113, #4225, #8537, #9822 ) ) ;
#1900=SURFACE_STYLE_USAGE ( .BOTH. , #9368 ) ;
#1903=DIRECTION ( 'NONE',  ( 0.000000000000000000, 0.000000000000000000, 1.000000000000000000 ) ) ;
#1904=DIRECTION ( 'NONE',  ( 0.000000000000000000, 1.000000000000000000, 0.000000000000000000 ) ) ;
#1918=CARTESIAN_POINT ( 'NONE',  ( -69.85388127645428824, 77.76794919243110371, 3.330127018922237614 ) ) ;
#1932=AXIS2_PLACEMENT_3D ( 'NONE', #5152, #8871, #3211 ) ;
#1939=DIRECTION ( 'NONE',  ( 0.000000000000000000, -0.8660254037844407060, 0.4999999999999965028 ) ) ;
#1947=EDGE_LOOP ( 'NONE', ( #4493, #4209, #2967, #5069 ) ) ;
#1957=CIRCLE ( 'NONE', #2153, 15.00000000000000000 ) ;
#1985=STYLED_ITEM ( 'NONE', ( #11194 ), #4372 ) ;
#2011=DIRECTION ( 'NONE',  ( 0.000000000000000000, 0.000000000000000000, 1.000000000000000000 ) ) ;
#2019=EDGE_CURVE ( 'NONE', #5470, #8579, #11159, .T. ) ;
#2033=CARTESIAN_POINT ( 'NONE',  ( -30.25776724459628753, 76.75431408359612817, 5.085794527760020500 ) ) ;
#2040=DIRECTION ( 'NONE',  ( 0.000000000000000000, 0.4999999999999962808, 0.8660254037844407060 ) ) ;
#2041=( BOUNDED_SURFACE ( )  B_SPLINE_SURFACE ( 3, 2, ( 
 ( #422, #4344, #6287 ),
 ( #8948, #3423, #2353 ),
 ( #614, #3294, #7097 ),
 ( #9131, #3232, #6042 ) ),
 .UNSPECIFIED., .F., .F., .F. ) 
 B_SPLINE_SURFACE_WITH_KNOTS ( ( 4, 4 ),
 ( 3, 3 ),
 ( 0.08252307147638787699, 0.08572545668793386808 ),
 ( 0.000000000000000000, 1.000000000000000000 ),
 .UNSPECIFIED. ) 
 GEOMETRIC_REPRESENTATION_ITEM ( )  RATIONAL_B_SPLINE_SURFACE ( (
 ( 1.000000000000000000, 0.8237544710479146604, 1.000000000000000000),
 ( 1.000000000000000000, 0.8337078205039558654, 1.000000000000000000),
 ( 1.000000000000000000, 0.8426243553970736988, 1.000000000000000000),
 ( 1.000000000000000000, 0.8507194741069452615, 1.000000000000000000) ) ) 
 REPRESENTATION_ITEM ( '' )  SURFACE ( )  );
#2049=DIRECTION ( 'NONE',  ( 0.000000000000000000, 0.000000000000000000, -1.000000000000000000 ) ) ;
#2051=ORIENTED_EDGE ( 'NONE', *, *, #4623, .F. ) ;
#2061=CARTESIAN_POINT ( 'NONE',  ( 0.000000000000000000, 87.00000000000000000, 0.000000000000000000 ) ) ;
#2075=VECTOR ( 'NONE', #3237, 1000.000000000000000 ) ;
#2076=FACE_OUTER_BOUND ( 'NONE', #10289, .T. ) ;
#2085=EDGE_CURVE ( 'NONE', #4062, #4534, #5791, .T. ) ;
#2089=EDGE_LOOP ( 'NONE', ( #9140, #4210, #268, #10094 ) ) ;
#2095=VECTOR ( 'NONE', #1614, 1000.000000000000000 ) ;
#2105=DIRECTION ( 'NONE',  ( 0.000000000000000000, -0.8660254037844402619, -0.4999999999999975575 ) ) ;
#2114=CARTESIAN_POINT ( 'NONE',  ( -34.73110591274434000, 77.00000000000000000, 8.660254037844445918 ) ) ;
#2119=VERTEX_POINT ( 'NONE', #5837 ) ;
#2121=DIRECTION ( 'NONE',  ( -1.000000000000000000, 0.000000000000000000, 0.000000000000000000 ) ) ;
#2134=VERTEX_POINT ( 'NONE', #6706 ) ;
#2147=FACE_OUTER_BOUND ( 'NONE', #2962, .T. ) ;
#2153=AXIS2_PLACEMENT_3D ( 'NONE', #9084, #6545, #5305 ) ;
#2157=ORIENTED_EDGE ( 'NONE', *, *, #2279, .F. ) ;
#2173=ORIENTED_EDGE ( 'NONE', *, *, #3226, .F. ) ;
#2183=EDGE_CURVE ( 'NONE', #7236, #5974, #11966, .T. ) ;
#2186=CARTESIAN_POINT ( 'NONE',  ( 0.000000000000000000, 92.00000000000000000, 0.000000000000000000 ) ) ;
#2201=ORIENTED_EDGE ( 'NONE', *, *, #3226, .T. ) ;
#2203=AXIS2_PLACEMENT_3D ( 'NONE', #3595, #5413, #2656 ) ;
#2208=ORIENTED_EDGE ( 'NONE', *, *, #2759, .T. ) ;
#2218=ORIENTED_EDGE ( 'NONE', *, *, #5864, .T. ) ;
#2222=DIRECTION ( 'NONE',  ( -1.000000000000000000, 0.000000000000000000, 0.000000000000000000 ) ) ;
#2223=CARTESIAN_POINT ( 'NONE',  ( -27.33018067101282256, 87.00000000000000000, -12.37179148263487605 ) ) ;
#2224=DIRECTION ( 'NONE',  ( -1.000000000000000000, 0.000000000000000000, 0.000000000000000000 ) ) ;
#2229=CARTESIAN_POINT ( 'NONE',  ( 0.000000000000000000, 165.5000000000000000, 0.000000000000000000 ) ) ;
#2232=FACE_OUTER_BOUND ( 'NONE', #9916, .T. ) ;
#2233=EDGE_CURVE ( 'NONE', #7634, #1834, #7698, .T. ) ;
#2235=ORIENTED_EDGE ( 'NONE', *, *, #10451, .T. ) ;
#2264=VERTEX_POINT ( 'NONE', #7878 ) ;
#2266=CARTESIAN_POINT ( 'NONE',  ( 34.73110591274434000, 77.00000000000000000, -8.660254037844445918 ) ) ;
#2277=CIRCLE ( 'NONE', #1285, 25.50000000000000000 ) ;
#2279=EDGE_CURVE ( 'NONE', #3932, #7967, #5569, .T. ) ;
#2281=DIRECTION ( 'NONE',  ( 0.000000000000000000, 0.8660254037844405950, -0.4999999999999965028 ) ) ;
#2290=DIRECTION ( 'NONE',  ( 0.000000000000000000, 0.000000000000000000, -1.000000000000000000 ) ) ;
#2294=ORIENTED_EDGE ( 'NONE', *, *, #4258, .T. ) ;
#2297=CARTESIAN_POINT ( 'NONE',  ( 34.84121487603211875, 75.26794919243111792, -7.660254037844449471 ) ) ;
#2298=DIRECTION ( 'NONE',  ( 0.000000000000000000, 0.000000000000000000, 1.000000000000000000 ) ) ;
#2304=TOROIDAL_SURFACE ( 'NONE', #2708, 24.99999999999999645, 0.5000000000000004441 ) ;
#2309=CARTESIAN_POINT ( 'NONE',  ( 32.15778161310143446, 87.00000000000000000, 8.660254037844435260 ) ) ;
#2320=CARTESIAN_POINT ( 'NONE',  ( 3.061616997868382648E-15, 87.00000000000000000, -24.99999999999999645 ) ) ;
#2327=CARTESIAN_POINT ( 'NONE',  ( 30.00100000000000122, 75.26794919243111792, 7.660254037844449471 ) ) ;
#2330=DIRECTION ( 'NONE',  ( 0.000000000000000000, 0.8660254037844407060, -0.4999999999999965583 ) ) ;
#2339=CARTESIAN_POINT ( 'NONE',  ( -29.42287733398164207, 85.62135522733750292, -10.27237124600374685 ) ) ;
#2344=AXIS2_PLACEMENT_3D ( 'NONE', #4238, #3309, #1318 ) ;
#2353=CARTESIAN_POINT ( 'NONE',  ( 32.12519652190606223, 85.41823950547951938, 9.573483885149325801 ) ) ;
#2366=CARTESIAN_POINT ( 'NONE',  ( 29.32777202433393526, 87.43477800909943198, 9.413311639618298088 ) ) ;
#2374=DIRECTION ( 'NONE',  ( 0.000000000000000000, 0.000000000000000000, 1.000000000000000000 ) ) ;
#2399=CYLINDRICAL_SURFACE ( 'NONE', #5552, 5.000000000000000000 ) ;
#2401=CARTESIAN_POINT ( 'NONE',  ( -27.52813290908667909, 87.44182241851447657, -11.93450069589770202 ) ) ;
#2412=ADVANCED_FACE ( 'NONE', ( #7499 ), #1705, .T. ) ;
#2416=EDGE_LOOP ( 'NONE', ( #6778, #2617, #12291, #4175 ) ) ;
#2425=CARTESIAN_POINT ( 'NONE',  ( -31.23312648697675797, 87.04033007153444146, -8.730107770814976575 ) ) ;
#2429=DIRECTION ( 'NONE',  ( -1.000000000000000000, 0.000000000000000000, 0.000000000000000000 ) ) ;
#2431=EDGE_LOOP ( 'NONE', ( #7696, #7036, #9329, #5583 ) ) ;
#2453=ORIENTED_EDGE ( 'NONE', *, *, #6299, .T. ) ;
#2467=CARTESIAN_POINT ( 'NONE',  ( 0.000000000000000000, 170.0000000000000000, 0.000000000000000000 ) ) ;
#2469=LINE ( 'NONE', #10816, #7444 ) ;
#2483=CARTESIAN_POINT ( 'NONE',  ( -8.500000000000000000, 165.5000000000000000, -6.164414002968973350 ) ) ;
#2487=ORIENTED_EDGE ( 'NONE', *, *, #10672, .T. ) ;
#2492=CARTESIAN_POINT ( 'NONE',  ( 2.143131898507868248E-15, 87.50000000000000000, 17.50000000000000000 ) ) ;
#2498=ORIENTED_EDGE ( 'NONE', *, *, #6710, .T. ) ;
#2506=CARTESIAN_POINT ( 'NONE',  ( 69.85388127645428824, 77.76794919243110371, -3.330127018922237614 ) ) ;
#2508=VERTEX_POINT ( 'NONE', #10293 ) ;
#2518=( BOUNDED_CURVE ( )  B_SPLINE_CURVE ( 3, ( #2803, #3521, #7324, #11123 ),
 .UNSPECIFIED., .F., .F. ) 
 B_SPLINE_CURVE_WITH_KNOTS ( ( 4, 4 ),
 ( 4.419546208656112363, 5.005231752113266985 ),
 .UNSPECIFIED. ) 
 CURVE ( )  GEOMETRIC_REPRESENTATION_ITEM ( )  RATIONAL_B_SPLINE_CURVE ( ( 1.000000000000000000, 0.9716180718375584391, 0.9716180718375584391, 1.000000000000000000 ) ) 
 REPRESENTATION_ITEM ( '' )  );
#2519=EDGE_LOOP ( 'NONE', ( #3043, #898, #6208, #10217 ) ) ;
#2523=DIRECTION ( 'NONE',  ( -0.000000000000000000, 1.000000000000000000, -0.000000000000000000 ) ) ;
#2529=EDGE_LOOP ( 'NONE', ( #10134, #941, #10729, #6130, #6110, #9810, #9335, #11430, #3942 ) ) ;
#2531=CARTESIAN_POINT ( 'NONE',  ( -32.05000697088088657, 85.26794919243110371, -9.660254037844429931 ) ) ;
#2534=CARTESIAN_POINT ( 'NONE',  ( -27.96269517408193295, 86.23182228119658532, -11.42938571145656113 ) ) ;
#2558=DIRECTION ( 'NONE',  ( 1.000000000000000000, -0.000000000000000000, 1.224646799147353207E-16 ) ) ;
#2559=CARTESIAN_POINT ( 'NONE',  ( -34.77127485704751564, 76.44489695195846934, 8.339765143629700006 ) ) ;
#2568=CARTESIAN_POINT ( 'NONE',  ( 27.67899820261485999, 88.38261385519929547, 11.05501148229834030 ) ) ;
#2591=AXIS2_PLACEMENT_3D ( 'NONE', #12353, #11489, #59 ) ;
#2593=CARTESIAN_POINT ( 'NONE',  ( 69.85388127645425982, 77.00000000000000000, -8.660254037844445918 ) ) ;
#2610=EDGE_LOOP ( 'NONE', ( #10047, #6944, #9511, #1873 ) ) ;
#2616=CARTESIAN_POINT ( 'NONE',  ( 1.285879139104720633E-15, 122.5000000000000000, 10.49999999999999822 ) ) ;
#2617=ORIENTED_EDGE ( 'NONE', *, *, #2746, .T. ) ;
#2621=AXIS2_PLACEMENT_3D ( 'NONE', #6498, #2684, #12234 ) ;
#2625=DIRECTION ( 'NONE',  ( -0.000000000000000000, -1.000000000000000000, -0.000000000000000000 ) ) ;
#2627=DIRECTION ( 'NONE',  ( 0.000000000000000000, 1.000000000000000000, 0.000000000000000000 ) ) ;
#2632=ADVANCED_FACE ( 'NONE', ( #955, #1879 ), #7676, .F. ) ;
#2640=FACE_OUTER_BOUND ( 'NONE', #2416, .T. ) ;
#2645=CIRCLE ( 'NONE', #6630, 17.00000000000000000 ) ;
#2649=CARTESIAN_POINT ( 'NONE',  ( -32.15133482848810331, 77.00000000000000000, 7.827692000169491848 ) ) ;
#2655=AXIS2_PLACEMENT_3D ( 'NONE', #11585, #10574, #2040 ) ;
#2656=DIRECTION ( 'NONE',  ( 0.000000000000000000, 0.000000000000000000, -1.000000000000000000 ) ) ;
#2662=VECTOR ( 'NONE', #7873, 1000.000000000000000 ) ;
#2666=ORIENTED_EDGE ( 'NONE', *, *, #8899, .T. ) ;
#2669=EDGE_LOOP ( 'NONE', ( #6979, #8099, #1828, #6259 ) ) ;
#2674=CARTESIAN_POINT ( 'NONE',  ( 0.000000000000000000, 165.5000000000000000, 0.000000000000000000 ) ) ;
#2683=AXIS2_PLACEMENT_3D ( 'NONE', #10168, #1642, #5449 ) ;
#2684=DIRECTION ( 'NONE',  ( 0.000000000000000000, -0.4999999999999965028, -0.8660254037844407060 ) ) ;
#2708=AXIS2_PLACEMENT_3D ( 'NONE', #5329, #9170, #11185 ) ;
#2724=ORIENTED_EDGE ( 'NONE', *, *, #7617, .F. ) ;
#2729=DIRECTION ( 'NONE',  ( 0.000000000000000000, 1.000000000000000000, 0.000000000000000000 ) ) ;
#2740=ORIENTED_EDGE ( 'NONE', *, *, #9346, .T. ) ;
#2742=DIRECTION ( 'NONE',  ( -0.000000000000000000, 0.4999999999999965028, 0.8660254037844407060 ) ) ;
#2746=EDGE_CURVE ( 'NONE', #5955, #11632, #8787, .T. ) ;
#2751=VECTOR ( 'NONE', #12258, 1000.000000000000000 ) ;
#2759=EDGE_CURVE ( 'NONE', #2264, #334, #11255, .T. ) ;
#2764=ORIENTED_EDGE ( 'NONE', *, *, #1822, .F. ) ;
#2765=( NAMED_UNIT ( * ) PLANE_ANGLE_UNIT ( ) SI_UNIT ( $, .RADIAN. ) );
#2766=EDGE_CURVE ( 'NONE', #1112, #11439, #1439, .T. ) ;
#2771=AXIS2_PLACEMENT_3D ( 'NONE', #10562, #4768, #24 ) ;
#2775=B_SPLINE_CURVE_WITH_KNOTS ( 'NONE', 3,
 ( #1617, #6538, #6352, #10325 ),
 .UNSPECIFIED., .F., .F.,
 ( 4, 4 ),
 ( 0.000000000000000000, 0.001357209897699809299 ),
 .UNSPECIFIED. ) ;
#2787=EDGE_CURVE ( 'NONE', #10587, #5507, #5939, .T. ) ;
#2790=PRODUCT_DEFINITION_SHAPE ( 'NONE', 'NONE',  #545 ) ;
#2800=FACE_OUTER_BOUND ( 'NONE', #2529, .T. ) ;
#2803=CARTESIAN_POINT ( 'NONE',  ( -28.72281323269012887, 87.00000000000000000, -8.660254037844435260 ) ) ;
#2806=EDGE_CURVE ( 'NONE', #2508, #945, #10970, .T. ) ;
#2809=CARTESIAN_POINT ( 'NONE',  ( -31.88521078284829713, 86.99999999999998579, -14.43375672974068991 ) ) ;
#2830=ADVANCED_FACE ( 'NONE', ( #6928 ), #10724, .F. ) ;
#2833=ORIENTED_EDGE ( 'NONE', *, *, #1657, .F. ) ;
#2841=( BOUNDED_CURVE ( )  B_SPLINE_CURVE ( 3, ( #8964, #1746, #3616, #3799 ),
 .UNSPECIFIED., .F., .F. ) 
 B_SPLINE_CURVE_WITH_KNOTS ( ( 4, 4 ),
 ( 4.419546208656112363, 5.005231752113266985 ),
 .UNSPECIFIED. ) 
 CURVE ( )  GEOMETRIC_REPRESENTATION_ITEM ( )  RATIONAL_B_SPLINE_CURVE ( ( 1.000000000000000000, 0.9716180718375584391, 0.9716180718375584391, 1.000000000000000000 ) ) 
 REPRESENTATION_ITEM ( '' )  );
#2844=EDGE_CURVE ( 'NONE', #4062, #7080, #11713, .T. ) ;
#2846=EDGE_CURVE ( 'NONE', #7525, #7634, #1957, .T. ) ;
#2853=EDGE_LOOP ( 'NONE', ( #3610, #6946, #1825, #10648 ) ) ;
#2856=CARTESIAN_POINT ( 'NONE',  ( 0.000000000000000000, 122.0000000000000000, 17.00000000000000000 ) ) ;
#2862=EDGE_LOOP ( 'NONE', ( #2918, #6840 ) ) ;
#2863=CARTESIAN_POINT ( 'NONE',  ( 30.98881549816775660, 77.00000000000001421, -6.657310619789788220 ) ) ;
#2883=ORIENTED_EDGE ( 'NONE', *, *, #10339, .T. ) ;
#2888=EDGE_CURVE ( 'NONE', #8670, #4839, #1756, .T. ) ;
#2903=CARTESIAN_POINT ( 'NONE',  ( -32.32195836398363298, 75.59155356138302295, 7.099754829268524858 ) ) ;
#2910=VECTOR ( 'NONE', #4647, 1000.000000000000000 ) ;
#2915=ADVANCED_FACE ( 'NONE', ( #10085 ), #11031, .T. ) ;
#2918=ORIENTED_EDGE ( 'NONE', *, *, #4353, .T. ) ;
#2927=DIRECTION ( 'NONE',  ( 0.000000000000000000, 1.000000000000000000, 0.000000000000000000 ) ) ;
#2948=ORIENTED_EDGE ( 'NONE', *, *, #4601, .T. ) ;
#2958=VECTOR ( 'NONE', #3371, 1000.000000000000000 ) ;
#2962=EDGE_LOOP ( 'NONE', ( #76, #10415 ) ) ;
#2963=DIRECTION ( 'NONE',  ( 0.000000000000000000, 0.000000000000000000, 1.000000000000000000 ) ) ;
#2967=ORIENTED_EDGE ( 'NONE', *, *, #10354, .T. ) ;
#2968=ORIENTED_EDGE ( 'NONE', *, *, #2806, .F. ) ;
#2970=EDGE_CURVE ( 'NONE', #3368, #6910, #556, .T. ) ;
#2974=EDGE_CURVE ( 'NONE', #8555, #7080, #10511, .T. ) ;
#2975=EDGE_CURVE ( 'NONE', #11714, #7098, #7526, .T. ) ;
#2980=CARTESIAN_POINT ( 'NONE',  ( -32.14616437604218646, 85.84037417286381810, -9.329764321300741514 ) ) ;
#2988=VECTOR ( 'NONE', #703, 1000.000000000000000 ) ;
#3025=CARTESIAN_POINT ( 'NONE',  ( 0.000000000000000000, 165.5000000000000000, 2.649999999999993694 ) ) ;
#3028=LINE ( 'NONE', #9682, #8873 ) ;
#3030=ORIENTED_EDGE ( 'NONE', *, *, #408, .F. ) ;
#3031=ORIENTED_EDGE ( 'NONE', *, *, #4877, .F. ) ;
#3033=ORIENTED_EDGE ( 'NONE', *, *, #6455, .T. ) ;
#3035=CARTESIAN_POINT ( 'NONE',  ( 0.000000000000000000, 92.00000000000000000, 24.99999999999999645 ) ) ;
#3036=DIRECTION ( 'NONE',  ( 0.000000000000000000, 1.000000000000000000, 0.000000000000000000 ) ) ;
#3042=AXIS2_PLACEMENT_3D ( 'NONE', #7697, #913, #6827 ) ;
#3043=ORIENTED_EDGE ( 'NONE', *, *, #6726, .F. ) ;
#3048=TOROIDAL_SURFACE ( 'NONE', #11820, 24.99999999999999645, 0.5000000000000004441 ) ;
#3070=VECTOR ( 'NONE', #5085, 1000.000000000000000 ) ;
#3073=EDGE_CURVE ( 'NONE', #10304, #11439, #7914, .T. ) ;
#3074=FACE_OUTER_BOUND ( 'NONE', #426, .T. ) ;
#3090=TOROIDAL_SURFACE ( 'NONE', #7477, 17.00000000000000000, 0.5000000000000004441 ) ;
#3093=VECTOR ( 'NONE', #6841, 1000.000000000000000 ) ;
#3106=CYLINDRICAL_SURFACE ( 'NONE', #813, 30.00000000000000000 ) ;
#3110=CARTESIAN_POINT ( 'NONE',  ( -73.35315233757310693, 81.28571428571424917, 1.237179148263527928 ) ) ;
#3126=CARTESIAN_POINT ( 'NONE',  ( 0.000000000000000000, 127.0000000000000000, -17.50000000000000000 ) ) ;
#3133=DIRECTION ( 'NONE',  ( 0.000000000000000000, -0.8660254037844401509, 0.4999999999999974465 ) ) ;
#3134=CARTESIAN_POINT ( 'NONE',  ( -27.30107202361637775, 86.87046582918780757, -12.43589427268144831 ) ) ;
#3135=CARTESIAN_POINT ( 'NONE',  ( -34.84121487603211875, 75.26794919243111792, 7.660254037844449471 ) ) ;
#3142=PRODUCT_DEFINITION_CONTEXT ( 'detailed design', #397, 'design' ) ;
#3143=LINE ( 'NONE', #8684, #2662 ) ;
#3158=DIRECTION ( 'NONE',  ( 0.000000000000000000, 1.000000000000000000, 0.000000000000000000 ) ) ;
#3177=CARTESIAN_POINT ( 'NONE',  ( -29.14112381217239900, 87.50172632198250255, -9.529269519012833811 ) ) ;
#3180=CIRCLE ( 'NONE', #9739, 0.5000000000000004441 ) ;
#3186=CARTESIAN_POINT ( 'NONE',  ( 27.88763417807735578, 88.17431669512683357, 10.69423021798056084 ) ) ;
#3195=DIRECTION ( 'NONE',  ( -0.000000000000000000, -1.000000000000000000, -0.000000000000000000 ) ) ;
#3201=VECTOR ( 'NONE', #721, 1000.000000000000000 ) ;
#3211=DIRECTION ( 'NONE',  ( 0.000000000000000000, 0.000000000000000000, 1.000000000000000000 ) ) ;
#3214=CIRCLE ( 'NONE', #7400, 25.50000000000000000 ) ;
#3216=VERTEX_POINT ( 'NONE', #1183 ) ;
#3220=AXIS2_PLACEMENT_3D ( 'NONE', #536, #7211, #8260 ) ;
#3226=EDGE_CURVE ( 'NONE', #80, #10035, #11498, .T. ) ;
#3227=ADVANCED_FACE ( 'NONE', ( #10940 ), #2399, .T. ) ;
#3231=VERTEX_POINT ( 'NONE', #3110 ) ;
#3232=CARTESIAN_POINT ( 'NONE',  ( 29.05832229253450549, 87.09380371750550864, 8.606096436291641893 ) ) ;
#3237=DIRECTION ( 'NONE',  ( -0.000000000000000000, -1.000000000000000000, -0.000000000000000000 ) ) ;
#3238=CARTESIAN_POINT ( 'NONE',  ( -28.78580657183879765, 87.64875042622799128, -9.783922737503317535 ) ) ;
#3245=CARTESIAN_POINT ( 'NONE',  ( 3.245314017740474622E-16, 170.0000000000000000, -2.649999999999987477 ) ) ;
#3258=CARTESIAN_POINT ( 'NONE',  ( -30.00100000000000122, 85.26794919243110371, 9.660254037844429931 ) ) ;
#3273=VECTOR ( 'NONE', #10824, 1000.000000000000000 ) ;
#3281=LINE ( 'NONE', #1413, #302 ) ;
#3294=CARTESIAN_POINT ( 'NONE',  ( 29.00531465893917371, 86.42397445337759621, 8.992822542244239159 ) ) ;
#3309=DIRECTION ( 'NONE',  ( 0.000000000000000000, 1.000000000000000000, 0.000000000000000000 ) ) ;
#3327=ORIENTED_EDGE ( 'NONE', *, *, #11690, .T. ) ;
#3334=EDGE_CURVE ( 'NONE', #4135, #10304, #3586, .T. ) ;
#3335=DIRECTION ( 'NONE',  ( 0.000000000000000000, 1.000000000000000000, 0.000000000000000000 ) ) ;
#3349=AXIS2_PLACEMENT_3D ( 'NONE', #10588, #2927, #10524 ) ;
#3366=CARTESIAN_POINT ( 'NONE',  ( 27.32050286291078933, 86.95679894682506017, 12.39317045950328300 ) ) ;
#3367=CARTESIAN_POINT ( 'NONE',  ( -28.61611180472258553, 87.72948999988449259, -9.923767781257849308 ) ) ;
#3368=VERTEX_POINT ( 'NONE', #7573 ) ;
#3371=DIRECTION ( 'NONE',  ( -0.000000000000000000, -1.000000000000000000, -0.000000000000000000 ) ) ;
#3394=ORIENTED_EDGE ( 'NONE', *, *, #1836, .T. ) ;
#3405=UNCERTAINTY_MEASURE_WITH_UNIT (LENGTH_MEASURE( 1.000000000000000082E-05 ), #8494, 'distance_accuracy_value', 'NONE');
#3412=CARTESIAN_POINT ( 'NONE',  ( 31.68100721119781937, 75.82462385531685811, -6.696065238440062295 ) ) ;
#3423=CARTESIAN_POINT ( 'NONE',  ( 28.82113438502227609, 85.77482169911409926, 9.367611059682538155 ) ) ;
#3428=AXIS2_PLACEMENT_3D ( 'NONE', #8939, #7829, #5039 ) ;
#3438=DIRECTION ( 'NONE',  ( 0.000000000000000000, 0.000000000000000000, 1.000000000000000000 ) ) ;
#3447=DIRECTION ( 'NONE',  ( -0.000000000000000000, -1.000000000000000000, -0.000000000000000000 ) ) ;
#3461=EDGE_LOOP ( 'NONE', ( #10813, #8441, #1881 ) ) ;
#3466=FACE_OUTER_BOUND ( 'NONE', #1897, .T. ) ;
#3485=ADVANCED_FACE ( 'NONE', ( #2147, #7695 ), #8622, .T. ) ;
#3494=DIRECTION ( 'NONE',  ( 0.000000000000000000, -0.000000000000000000, 1.000000000000000000 ) ) ;
#3503=DIRECTION ( 'NONE',  ( -0.000000000000000000, -1.000000000000000000, -0.000000000000000000 ) ) ;
#3507=EDGE_LOOP ( 'NONE', ( #7921, #2157 ) ) ;
#3515=EDGE_CURVE ( 'NONE', #9969, #9385, #8064, .T. ) ;
#3520=ORIENTED_EDGE ( 'NONE', *, *, #2888, .T. ) ;
#3521=CARTESIAN_POINT ( 'NONE',  ( -30.43816488677641630, 83.71535165408627677, -2.971076217724753832 ) ) ;
#3526=ORIENTED_EDGE ( 'NONE', *, *, #248, .F. ) ;
#3529=FACE_OUTER_BOUND ( 'NONE', #10150, .T. ) ;
#3530=CARTESIAN_POINT ( 'NONE',  ( -30.50145854323920602, 85.38003226577613702, -9.854387615546507107 ) ) ;
#3532=DIRECTION ( 'NONE',  ( 0.000000000000000000, -0.8660254037844402619, 0.4999999999999975575 ) ) ;
#3543=DIRECTION ( 'NONE',  ( 0.000000000000000000, 0.000000000000000000, -1.000000000000000000 ) ) ;
#3544=DIRECTION ( 'NONE',  ( 0.000000000000000000, 1.000000000000000000, 0.000000000000000000 ) ) ;
#3553=CARTESIAN_POINT ( 'NONE',  ( 34.84179752789421514, 75.25738092153642356, -7.654152443798540872 ) ) ;
#3564=FACE_BOUND ( 'NONE', #7875, .T. ) ;
#3565=ORIENTED_EDGE ( 'NONE', *, *, #4744, .T. ) ;
#3569=ORIENTED_EDGE ( 'NONE', *, *, #2183, .T. ) ;
#3586=LINE ( 'NONE', #1837, #2751 ) ;
#3594=AXIS2_PLACEMENT_3D ( 'NONE', #6723, #4158, #2290 ) ;
#3595=CARTESIAN_POINT ( 'NONE',  ( 0.000000000000000000, 216.0365690573663926, 0.000000000000000000 ) ) ;
#3596=AXIS2_PLACEMENT_3D ( 'NONE', #5590, #1904, #4835 ) ;
#3609=EDGE_CURVE ( 'NONE', #4534, #4062, #5705, .T. ) ;
#3610=ORIENTED_EDGE ( 'NONE', *, *, #11582, .F. ) ;
#3613=ORIENTED_EDGE ( 'NONE', *, *, #1071, .T. ) ;
#3616=CARTESIAN_POINT ( 'NONE',  ( 30.43816488677641985, 80.28464834591375165, -2.971076217724743618 ) ) ;
#3640=EDGE_CURVE ( 'NONE', #11487, #5761, #722, .T. ) ;
#3651=ADVANCED_FACE ( 'NONE', ( #12125 ), #1827, .F. ) ;
#3652=CARTESIAN_POINT ( 'NONE',  ( -27.54203853141981995, 86.50063778822037364, -11.90690952824024329 ) ) ;
#3668=ORIENTED_EDGE ( 'NONE', *, *, #9330, .F. ) ;
#3676=CARTESIAN_POINT ( 'NONE',  ( 0.000000000000000000, 87.50000000000000000, 0.000000000000000000 ) ) ;
#3677=DIRECTION ( 'NONE',  ( 0.000000000000000000, 0.000000000000000000, 1.000000000000000000 ) ) ;
#3688=CIRCLE ( 'NONE', #1106, 10.49999999999999822 ) ;
#3736=DIRECTION ( 'NONE',  ( -0.000000000000000000, 0.8660254037844402619, -0.4999999999999975575 ) ) ;
#3737=EDGE_LOOP ( 'NONE', ( #9152, #11526 ) ) ;
#3741=DIRECTION ( 'NONE',  ( -0.000000000000000000, -1.000000000000000000, -0.000000000000000000 ) ) ;
#3754=DIRECTION ( 'NONE',  ( 0.000000000000000000, -0.8660254037844402619, -0.4999999999999975575 ) ) ;
#3761=CARTESIAN_POINT ( 'NONE',  ( -32.05000697088088657, 85.26794919243110371, -9.660254037844429931 ) ) ;
#3769=DIRECTION ( 'NONE',  ( 0.000000000000000000, 1.000000000000000000, 0.000000000000000000 ) ) ;
#3770=CIRCLE ( 'NONE', #6956, 2.649999999999987477 ) ;
#3783=CARTESIAN_POINT ( 'NONE',  ( 27.96741528345890870, 86.27927944434865992, 11.41192941739706335 ) ) ;
#3797=VERTEX_POINT ( 'NONE', #10607 ) ;
#3799=CARTESIAN_POINT ( 'NONE',  ( 28.72281323269012532, 77.00000000000000000, -8.660254037844445918 ) ) ;
#3800=ORIENTED_EDGE ( 'NONE', *, *, #973, .T. ) ;
#3813=AXIS2_PLACEMENT_3D ( 'NONE', #12043, #6493, #691 ) ;
#3817=DIRECTION ( 'NONE',  ( 0.000000000000000000, 1.000000000000000000, 0.000000000000000000 ) ) ;
#3823=EDGE_CURVE ( 'NONE', #8953, #7769, #5760, .T. ) ;
#3834=SURFACE_STYLE_FILL_AREA ( #11446 ) ;
#3837=ORIENTED_EDGE ( 'NONE', *, *, #7456, .T. ) ;
#3840=CARTESIAN_POINT ( 'NONE',  ( -31.68100721119781937, 75.82462385531685811, 6.696065238440062295 ) ) ;
#3848=FACE_OUTER_BOUND ( 'NONE', #11983, .T. ) ;
#3865=CARTESIAN_POINT ( 'NONE',  ( 30.23169114332096896, 76.99999999999998579, -5.192055827170280580 ) ) ;
#3867=ORIENTED_EDGE ( 'NONE', *, *, #6315, .T. ) ;
#3890=CARTESIAN_POINT ( 'NONE',  ( -27.96741528345882344, 86.27927944434871677, -11.41192941739715927 ) ) ;
#3916=DIRECTION ( 'NONE',  ( 0.000000000000000000, 1.000000000000000000, 0.000000000000000000 ) ) ;
#3932=VERTEX_POINT ( 'NONE', #11734 ) ;
#3942=ORIENTED_EDGE ( 'NONE', *, *, #5719, .T. ) ;
#3963=CARTESIAN_POINT ( 'NONE',  ( -32.78711330112231792, 75.47285661897714704, 7.305343964218459440 ) ) ;
#3970=CARTESIAN_POINT ( 'NONE',  ( 28.48065962374913695, 85.97961707684491728, 10.89289897176416666 ) ) ;
#3989=CARTESIAN_POINT ( 'NONE',  ( 27.96269517408201821, 86.23182228119654269, 11.42938571145646875 ) ) ;
#3990=EDGE_LOOP ( 'NONE', ( #10978, #1858, #1559, #8988 ) ) ;
#3991=ADVANCED_FACE ( 'NONE', ( #10216 ), #7038, .T. ) ;
#3999=ORIENTED_EDGE ( 'NONE', *, *, #4145, .T. ) ;
#4003=CARTESIAN_POINT ( 'NONE',  ( -13.00000000000000178, 170.0000000000000000, -7.483314773547880883 ) ) ;
#4008=PLANE ( 'NONE',  #1732 ) ;
#4012=CIRCLE ( 'NONE', #4403, 5.000000000000000888 ) ;
#4016=EDGE_CURVE ( 'NONE', #4117, #8618, #1720, .T. ) ;
#4027=CARTESIAN_POINT ( 'NONE',  ( -30.49437064397536901, 76.52118294276679933, 5.489589508502957571 ) ) ;
#4029=EDGE_LOOP ( 'NONE', ( #8804, #4229, #9177, #1653, #10623, #205, #5758, #3565 ) ) ;
#4032=EDGE_CURVE ( 'NONE', #5307, #10772, #11206, .T. ) ;
#4033=FACE_OUTER_BOUND ( 'NONE', #2610, .T. ) ;
#4051=ORIENTED_EDGE ( 'NONE', *, *, #3073, .F. ) ;
#4062=VERTEX_POINT ( 'NONE', #5801 ) ;
#4073=DIRECTION ( 'NONE',  ( 0.000000000000000000, 0.000000000000000000, 1.000000000000000000 ) ) ;
#4116=( BOUNDED_CURVE ( )  B_SPLINE_CURVE ( 3, ( #2297, #9769, #7899, #1364 ),
 .UNSPECIFIED., .F., .F. ) 
 B_SPLINE_CURVE_WITH_KNOTS ( ( 4, 4 ),
 ( 1.666086958916892291, 1.694832046014206117 ),
 .UNSPECIFIED. ) 
 CURVE ( )  GEOMETRIC_REPRESENTATION_ITEM ( )  RATIONAL_B_SPLINE_CURVE ( ( 1.000000000000000000, 0.9999311445159493328, 0.9999311445159493328, 1.000000000000000000 ) ) 
 REPRESENTATION_ITEM ( '' )  );
#4117=VERTEX_POINT ( 'NONE', #1003 ) ;
#4121=CARTESIAN_POINT ( 'NONE',  ( 29.71888078761409346, 87.31388704012290702, 9.203922339174773981 ) ) ;
#4124=DIRECTION ( 'NONE',  ( -0.000000000000000000, -1.000000000000000000, -0.000000000000000000 ) ) ;
#4130=ORIENTED_EDGE ( 'NONE', *, *, #2970, .T. ) ;
#4135=VERTEX_POINT ( 'NONE', #7725 ) ;
#4145=EDGE_CURVE ( 'NONE', #945, #931, #330, .T. ) ;
#4157=ORIENTED_EDGE ( 'NONE', *, *, #5520, .T. ) ;
#4158=DIRECTION ( 'NONE',  ( -0.000000000000000000, -1.000000000000000000, -0.000000000000000000 ) ) ;
#4160=ORIENTED_EDGE ( 'NONE', *, *, #7644, .T. ) ;
#4171=CARTESIAN_POINT ( 'NONE',  ( -29.71888078761410767, 87.31388704012290702, -9.203922339174775757 ) ) ;
#4175=ORIENTED_EDGE ( 'NONE', *, *, #4419, .F. ) ;
#4187=CARTESIAN_POINT ( 'NONE',  ( 0.000000000000000000, 92.00000000000000000, 0.000000000000000000 ) ) ;
#4207=AXIS2_PLACEMENT_3D ( 'NONE', #1918, #2105, #9570 ) ;
#4209=ORIENTED_EDGE ( 'NONE', *, *, #3515, .T. ) ;
#4210=ORIENTED_EDGE ( 'NONE', *, *, #2844, .T. ) ;
#4220=CARTESIAN_POINT ( 'NONE',  ( 3.367778697655220913E-15, 92.00000000000000000, -24.99999999999999645 ) ) ;
#4225=ORIENTED_EDGE ( 'NONE', *, *, #7597, .T. ) ;
#4226=DIRECTION ( 'NONE',  ( 0.000000000000000000, 0.000000000000000000, 1.000000000000000000 ) ) ;
#4229=ORIENTED_EDGE ( 'NONE', *, *, #6676, .T. ) ;
#4231=LINE ( 'NONE', #10778, #2075 ) ;
#4234=CIRCLE ( 'NONE', #11217, 5.000000000000000000 ) ;
#4236=ADVANCED_FACE ( 'NONE', ( #2232 ), #9893, .T. ) ;
#4238=CARTESIAN_POINT ( 'NONE',  ( 0.000000000000000000, 170.0000000000000000, 0.000000000000000000 ) ) ;
#4249=CARTESIAN_POINT ( 'NONE',  ( 28.12254474901590484, 87.93978760833334718, 10.28801392380147206 ) ) ;
#4258=EDGE_CURVE ( 'NONE', #10229, #945, #4116, .T. ) ;
#4276=CIRCLE ( 'NONE', #8046, 2.649999999999993694 ) ;
#4277=CARTESIAN_POINT ( 'NONE',  ( -27.67899820261485999, 88.38261385519929547, -11.05501148229834030 ) ) ;
#4290=EDGE_CURVE ( 'NONE', #7703, #10799, #4276, .T. ) ;
#4299=EDGE_LOOP ( 'NONE', ( #7130, #2764, #4727, #2173, #1393 ) ) ;
#4300=DIRECTION ( 'NONE',  ( 1.000000000000000000, 0.000000000000000000, 0.000000000000000000 ) ) ;
#4303=TOROIDAL_SURFACE ( 'NONE', #6700, 24.99999999999999645, 5.000000000000000000 ) ;
#4304=DIRECTION ( 'NONE',  ( 1.224646799147353454E-16, 0.000000000000000000, -1.000000000000000000 ) ) ;
#4307=CARTESIAN_POINT ( 'NONE',  ( 0.000000000000000000, 127.0000000000000000, 0.000000000000000000 ) ) ;
#4327=DIRECTION ( 'NONE',  ( 0.000000000000000000, -0.000000000000000000, 1.000000000000000000 ) ) ;
#4330=CARTESIAN_POINT ( 'NONE',  ( 30.55518048406710818, 80.37544454677752981, 1.186187415305626436 ) ) ;
#4341=EDGE_CURVE ( 'NONE', #11487, #3231, #11282, .T. ) ;
#4344=CARTESIAN_POINT ( 'NONE',  ( 28.52887280570638495, 85.15789473684209554, 9.723794007404251261 ) ) ;
#4346=DIRECTION ( 'NONE',  ( 0.000000000000000000, 0.000000000000000000, 1.000000000000000000 ) ) ;
#4353=EDGE_CURVE ( 'NONE', #7098, #11714, #11656, .T. ) ;
#4358=FACE_BOUND ( 'NONE', #9792, .T. ) ;
#4361=ORIENTED_EDGE ( 'NONE', *, *, #6169, .T. ) ;
#4364=VERTEX_POINT ( 'NONE', #9198 ) ;
#4368=ORIENTED_EDGE ( 'NONE', *, *, #408, .T. ) ;
#4372=ADVANCED_BREP_SHAPE_REPRESENTATION ( '', ( #763, #1612 ), #10102 ) ;
#4383=CARTESIAN_POINT ( 'NONE',  ( -27.30107202361637775, 86.87046582918780757, -12.43589427268144831 ) ) ;
#4389=EDGE_CURVE ( 'NONE', #945, #8618, #4597, .T. ) ;
#4394=CARTESIAN_POINT ( 'NONE',  ( -30.98881549816775660, 77.00000000000001421, 6.657310619789788220 ) ) ;
#4396=CARTESIAN_POINT ( 'NONE',  ( -32.21610632499845650, 86.34645847305816346, -9.037576414350890985 ) ) ;
#4398=CARTESIAN_POINT ( 'NONE',  ( 30.63265341208206038, 76.40790137508867019, -5.685798939282528330 ) ) ;
#4403=AXIS2_PLACEMENT_3D ( 'NONE', #9970, #2558, #4304 ) ;
#4405=EDGE_CURVE ( 'NONE', #7080, #8555, #10646, .T. ) ;
#4408=CARTESIAN_POINT ( 'NONE',  ( 28.72281323269012532, 87.00000000000000000, 8.660254037844435260 ) ) ;
#4419=EDGE_CURVE ( 'NONE', #6910, #4839, #11147, .T. ) ;
#4423=CARTESIAN_POINT ( 'NONE',  ( 30.03968734988933420, 77.39454232463201322, -4.824121477407818048 ) ) ;
#4424=DIRECTION ( 'NONE',  ( 0.000000000000000000, 1.000000000000000000, 0.000000000000000000 ) ) ;
#4426=FACE_OUTER_BOUND ( 'NONE', #9300, .T. ) ;
#4435=VECTOR ( 'NONE', #817, 1000.000000000000000 ) ;
#4453=FILL_AREA_STYLE ('',( #657 ) ) ;
#4455=FACE_BOUND ( 'NONE', #9008, .T. ) ;
#4456=CARTESIAN_POINT ( 'NONE',  ( -69.85388127645428824, 17.99999999999971223, -31.17691453623957543 ) ) ;
#4457=CARTESIAN_POINT ( 'NONE',  ( 0.000000000000000000, 127.0000000000000000, -15.00000000000000000 ) ) ;
#4460=CARTESIAN_POINT ( 'NONE',  ( 0.000000000000000000, 122.5000000000000000, -10.49999999999999822 ) ) ;
#4473=CARTESIAN_POINT ( 'NONE',  ( 0.000000000000000000, 216.0365690573663926, 0.000000000000000000 ) ) ;
#4475=LINE ( 'NONE', #1675, #10465 ) ;
#4477=LINE ( 'NONE', #7531, #6653 ) ;
#4481=ORIENTED_EDGE ( 'NONE', *, *, #2746, .F. ) ;
#4493=ORIENTED_EDGE ( 'NONE', *, *, #5646, .F. ) ;
#4494=ADVANCED_FACE ( 'NONE', ( #6289 ), #9133, .T. ) ;
#4499=DIRECTION ( 'NONE',  ( 0.000000000000000000, 1.000000000000000000, 0.000000000000000000 ) ) ;
#4505=AXIS2_PLACEMENT_3D ( 'NONE', #1293, #5104, #6216 ) ;
#4509=ORIENTED_EDGE ( 'NONE', *, *, #7456, .F. ) ;
#4511=CARTESIAN_POINT ( 'NONE',  ( 0.000000000000000000, 122.0000000000000000, 0.000000000000000000 ) ) ;
#4515=DIRECTION ( 'NONE',  ( 0.000000000000000000, 0.000000000000000000, 1.000000000000000000 ) ) ;
#4519=( NAMED_UNIT ( * ) PLANE_ANGLE_UNIT ( ) SI_UNIT ( $, .RADIAN. ) );
#4522=AXIS2_PLACEMENT_3D ( 'NONE', #8348, #4499, #8289 ) ;
#4528=DIRECTION ( 'NONE',  ( 0.000000000000000000, 1.000000000000000000, 0.000000000000000000 ) ) ;
#4532=CARTESIAN_POINT ( 'NONE',  ( -30.07733313487553772, 77.00000000000709122, 4.660254037819535178 ) ) ;
#4534=VERTEX_POINT ( 'NONE', #7650 ) ;
#4538=PLANE ( 'NONE',  #6265 ) ;
#4545=CARTESIAN_POINT ( 'NONE',  ( 34.72842983617974966, 77.03714026276665550, -8.681696978550554888 ) ) ;
#4547=VERTEX_POINT ( 'NONE', #6654 ) ;
#4556=DIRECTION ( 'NONE',  ( 0.000000000000000000, 1.000000000000000000, 0.000000000000000000 ) ) ;
#4562=ORIENTED_EDGE ( 'NONE', *, *, #8620, .F. ) ;
#4575=SURFACE_STYLE_FILL_AREA ( #4453 ) ;
#4584=CARTESIAN_POINT ( 'NONE',  ( -27.97213591028565460, 86.27509468223345834, -11.40681812415373209 ) ) ;
#4597=LINE ( 'NONE', #676, #1298 ) ;
#4599=ORIENTED_EDGE ( 'NONE', *, *, #10451, .F. ) ;
#4601=EDGE_CURVE ( 'NONE', #334, #2134, #9445, .T. ) ;
#4609=DIRECTION ( 'NONE',  ( 0.000000000000000000, 1.000000000000000000, 0.000000000000000000 ) ) ;
#4610=DIRECTION ( 'NONE',  ( -0.000000000000000000, 0.8660254037844402619, 0.4999999999999975575 ) ) ;
#4616=CARTESIAN_POINT ( 'NONE',  ( 0.000000000000000000, 87.00000000000000000, 0.000000000000000000 ) ) ;
#4617=FACE_OUTER_BOUND ( 'NONE', #10323, .T. ) ;
#4623=EDGE_CURVE ( 'NONE', #11632, #6660, #3688, .T. ) ;
#4640=B_SPLINE_CURVE_WITH_KNOTS ( 'NONE', 3,
 ( #1108, #4779, #226, #9753, #4914, #9569, #8697, #3970, #12333, #3783 ),
 .UNSPECIFIED., .F., .F.,
 ( 4, 2, 2, 2, 4 ),
 ( 2.797157557069881010E-17, 0.001173140257025584660, 0.002346280514051141131, 0.003519420771076697818, 0.004692561028102254506 ),
 .UNSPECIFIED. ) ;
#4647=DIRECTION ( 'NONE',  ( -0.000000000000000000, -1.000000000000000000, -0.000000000000000000 ) ) ;
#4655=ORIENTED_EDGE ( 'NONE', *, *, #2233, .T. ) ;
#4670=CARTESIAN_POINT ( 'NONE',  ( -69.85388127645428824, 79.49999999999998579, 4.330127018922231841 ) ) ;
#4677=CIRCLE ( 'NONE', #10647, 10.49999999999999822 ) ;
#4683=CIRCLE ( 'NONE', #6882, 17.00000000000000000 ) ;
#4688=CARTESIAN_POINT ( 'NONE',  ( 32.18413411689675030, 86.41755723128771649, 8.996527527148016290 ) ) ;
#4697=VECTOR ( 'NONE', #2121, 1000.000000000000000 ) ;
#4702=ORIENTED_EDGE ( 'NONE', *, *, #5259, .F. ) ;
#4718=CARTESIAN_POINT ( 'NONE',  ( 0.000000000000000000, 216.0365690573663926, 0.000000000000000000 ) ) ;
#4727=ORIENTED_EDGE ( 'NONE', *, *, #9593, .F. ) ;
#4729=CARTESIAN_POINT ( 'NONE',  ( -30.00100000000000122, 85.26794919243110371, 9.660254037844429931 ) ) ;
#4733=ORIENTED_EDGE ( 'NONE', *, *, #1822, .T. ) ;
#4739=MECHANICAL_DESIGN_GEOMETRIC_PRESENTATION_REPRESENTATION('',(#1985),#386);
#4744=EDGE_CURVE ( 'NONE', #4364, #7558, #3281, .T. ) ;
#4748=CARTESIAN_POINT ( 'NONE',  ( 0.000000000000000000, 87.50000000000000000, 0.000000000000000000 ) ) ;
#4755=CARTESIAN_POINT ( 'NONE',  ( 30.00100000000000122, 85.26794919243110371, -9.660254037844429931 ) ) ;
#4765=CARTESIAN_POINT ( 'NONE',  ( -13.00000000000000178, 127.0000000000000000, -7.483314773547880883 ) ) ;
#4768=DIRECTION ( 'NONE',  ( -0.000000000000000000, -1.000000000000000000, -0.000000000000000000 ) ) ;
#4779=CARTESIAN_POINT ( 'NONE',  ( 31.65330186654243505, 85.26794919243108950, 9.660254037844429931 ) ) ;
#4789=ADVANCED_FACE ( 'NONE', ( #228 ), #7538, .F. ) ;
#4790=AXIS2_PLACEMENT_3D ( 'NONE', #6816, #1084, #4073 ) ;
#4798=CARTESIAN_POINT ( 'NONE',  ( 33.64113847583112715, 77.00000000000000000, -8.529771698700599813 ) ) ;
#4805=DIRECTION ( 'NONE',  ( 0.000000000000000000, 0.000000000000000000, -1.000000000000000000 ) ) ;
#4811=CIRCLE ( 'NONE', #5414, 15.00000000000000000 ) ;
#4817=CARTESIAN_POINT ( 'NONE',  ( -30.00100000000000122, 77.00000000000000000, -4.660254037844413944 ) ) ;
#4825=DIRECTION ( 'NONE',  ( 0.000000000000000000, 0.000000000000000000, 1.000000000000000000 ) ) ;
#4835=DIRECTION ( 'NONE',  ( 0.000000000000000000, 0.000000000000000000, 1.000000000000000000 ) ) ;
#4839=VERTEX_POINT ( 'NONE', #7399 ) ;
#4846=DIRECTION ( 'NONE',  ( 0.000000000000000000, 0.000000000000000000, -1.000000000000000000 ) ) ;
#4852=CARTESIAN_POINT ( 'NONE',  ( -32.05000697088088657, 85.26794919243110371, -9.660254037844429931 ) ) ;
#4855=CARTESIAN_POINT ( 'NONE',  ( 0.000000000000000000, 92.00000000000000000, 0.000000000000000000 ) ) ;
#4858=ORIENTED_EDGE ( 'NONE', *, *, #1845, .F. ) ;
#4866=ADVANCED_FACE ( 'NONE', ( #5283 ), #9271, .F. ) ;
#4877=EDGE_CURVE ( 'NONE', #11869, #10169, #4683, .T. ) ;
#4886=ORIENTED_EDGE ( 'NONE', *, *, #3334, .T. ) ;
#4888=CARTESIAN_POINT ( 'NONE',  ( 32.15778161310143446, 87.00000000000000000, 8.660254037844435260 ) ) ;
#4903=CARTESIAN_POINT ( 'NONE',  ( 0.000000000000000000, 92.00000000000000000, 0.000000000000000000 ) ) ;
#4914=CARTESIAN_POINT ( 'NONE',  ( 30.12465603153684413, 85.44772375131799436, 9.971632707744760182 ) ) ;
#4927=ORIENTED_EDGE ( 'NONE', *, *, #9330, .T. ) ;
#4955=EDGE_CURVE ( 'NONE', #7513, #11122, #7683, .T. ) ;
#4966=ADVANCED_FACE ( 'NONE', ( #2076 ), #1203, .F. ) ;
#4981=ORIENTED_EDGE ( 'NONE', *, *, #4419, .T. ) ;
#4987=ORIENTED_EDGE ( 'NONE', *, *, #10117, .F. ) ;
#4988=CARTESIAN_POINT ( 'NONE',  ( 32.15133482848810331, 77.00000000000000000, -7.827692000169491848 ) ) ;
#4993=DIRECTION ( 'NONE',  ( 1.000000000000000000, 0.000000000000000000, 0.000000000000000000 ) ) ;
#4997=AXIS2_PLACEMENT_3D ( 'NONE', #2229, #6101, #9885 ) ;
#5000=DIRECTION ( 'NONE',  ( 0.000000000000000000, -0.000000000000000000, 1.000000000000000000 ) ) ;
#5006=AXIS2_PLACEMENT_3D ( 'NONE', #5629, #8416, #12240 ) ;
#5009=DIRECTION ( 'NONE',  ( 0.000000000000000000, 1.000000000000000000, 0.000000000000000000 ) ) ;
#5018=EDGE_LOOP ( 'NONE', ( #5058, #4702, #4886, #497 ) ) ;
#5023=CIRCLE ( 'NONE', #1831, 22.00000000000000355 ) ;
#5032=DIRECTION ( 'NONE',  ( 1.000000000000000000, 0.000000000000000000, 0.000000000000000000 ) ) ;
#5033=ORIENTED_EDGE ( 'NONE', *, *, #5221, .F. ) ;
#5039=DIRECTION ( 'NONE',  ( 0.000000000000000000, 0.000000000000000000, 1.000000000000000000 ) ) ;
#5054=CARTESIAN_POINT ( 'NONE',  ( 27.95322648060798087, 86.18856968700900723, 11.45194355884130388 ) ) ;
#5058=ORIENTED_EDGE ( 'NONE', *, *, #2766, .F. ) ;
#5062=AXIS2_PLACEMENT_3D ( 'NONE', #2467, #593, #8251 ) ;
#5069=ORIENTED_EDGE ( 'NONE', *, *, #10117, .T. ) ;
#5077=CARTESIAN_POINT ( 'NONE',  ( -34.77260134704101802, 76.42358343581042845, 8.327459779344241753 ) ) ;
#5079=CYLINDRICAL_SURFACE ( 'NONE', #11757, 30.00000000000000000 ) ;
#5085=DIRECTION ( 'NONE',  ( 0.000000000000000000, 0.8660254037844405950, -0.4999999999999965028 ) ) ;
#5092=AXIS2_PLACEMENT_3D ( 'NONE', #864, #929, #9383 ) ;
#5104=DIRECTION ( 'NONE',  ( -0.000000000000000000, 0.8660254037844402619, 0.4999999999999975575 ) ) ;
#5116=DIRECTION ( 'NONE',  ( 0.000000000000000000, 0.000000000000000000, -1.000000000000000000 ) ) ;
#5119=CARTESIAN_POINT ( 'NONE',  ( 0.000000000000000000, 170.0000000000000000, -15.00000000000000000 ) ) ;
#5137=CARTESIAN_POINT ( 'NONE',  ( -13.00000000000000178, 216.0365690573663926, -7.483314773547880883 ) ) ;
#5152=CARTESIAN_POINT ( 'NONE',  ( 0.000000000000000000, 122.0000000000000000, 0.000000000000000000 ) ) ;
#5165=ADVANCED_FACE ( 'NONE', ( #9216 ), #696, .F. ) ;
#5174=EDGE_LOOP ( 'NONE', ( #2666, #6583, #7377, #9828 ) ) ;
#5182=VECTOR ( 'NONE', #5441, 1000.000000000000000 ) ;
#5184=CARTESIAN_POINT ( 'NONE',  ( 30.34950626935405182, 87.16600977219414403, 8.947791397837656646 ) ) ;
#5189=ORIENTED_EDGE ( 'NONE', *, *, #11515, .F. ) ;
#5196=CARTESIAN_POINT ( 'NONE',  ( 69.85388127645428824, 75.26794919243114634, -7.660254037844465458 ) ) ;
#5208=DIRECTION ( 'NONE',  ( 0.000000000000000000, 0.4999999999999966138, 0.8660254037844407060 ) ) ;
#5209=DIRECTION ( 'NONE',  ( 0.000000000000000000, 1.000000000000000000, 0.000000000000000000 ) ) ;
#5215=ORIENTED_EDGE ( 'NONE', *, *, #638, .T. ) ;
#5221=EDGE_CURVE ( 'NONE', #3368, #8670, #5683, .T. ) ;
#5237=LINE ( 'NONE', #6977, #10037 ) ;
#5259=EDGE_CURVE ( 'NONE', #4135, #1112, #7077, .T. ) ;
#5262=DIRECTION ( 'NONE',  ( 0.000000000000000000, 0.000000000000000000, 1.000000000000000000 ) ) ;
#5275=ORIENTED_EDGE ( 'NONE', *, *, #8275, .T. ) ;
#5283=FACE_OUTER_BOUND ( 'NONE', #4299, .T. ) ;
#5296=CARTESIAN_POINT ( 'NONE',  ( 0.000000000000000000, 165.5000000000000000, 0.000000000000000000 ) ) ;
#5299=DIRECTION ( 'NONE',  ( 0.000000000000000000, 0.8660254037844405950, 0.4999999999999965028 ) ) ;
#5305=DIRECTION ( 'NONE',  ( 0.000000000000000000, 0.000000000000000000, 1.000000000000000000 ) ) ;
#5307=VERTEX_POINT ( 'NONE', #6496 ) ;
#5320=CIRCLE ( 'NONE', #1932, 22.00000000000000355 ) ;
#5329=CARTESIAN_POINT ( 'NONE',  ( 0.000000000000000000, 87.00000000000000000, 0.000000000000000000 ) ) ;
#5334=( NAMED_UNIT ( * ) PLANE_ANGLE_UNIT ( ) SI_UNIT ( $, .RADIAN. ) );
#5338=CARTESIAN_POINT ( 'NONE',  ( -34.73110591274434000, 77.00000000000000000, 8.660254037844445918 ) ) ;
#5365=CARTESIAN_POINT ( 'NONE',  ( 29.94260118448502794, 78.56931597186009242, -5.428213010295147356 ) ) ;
#5396=EDGE_LOOP ( 'NONE', ( #11610, #8502 ) ) ;
#5398=AXIS2_PLACEMENT_3D ( 'NONE', #12251, #8547, #784 ) ;
#5413=DIRECTION ( 'NONE',  ( -0.000000000000000000, -1.000000000000000000, -0.000000000000000000 ) ) ;
#5414=AXIS2_PLACEMENT_3D ( 'NONE', #1443, #8034, #7050 ) ;
#5425=EDGE_LOOP ( 'NONE', ( #7116, #7542, #10605, #802 ) ) ;
#5428=EDGE_LOOP ( 'NONE', ( #111, #10454, #2833, #647 ) ) ;
#5430=CARTESIAN_POINT ( 'NONE',  ( 30.99900678938364251, 76.83479030960515388, -8.564870178622241426 ) ) ;
#5431=CARTESIAN_POINT ( 'NONE',  ( 0.000000000000000000, 87.00000000000000000, 0.000000000000000000 ) ) ;
#5441=DIRECTION ( 'NONE',  ( 0.000000000000000000, -0.8660254037844405950, 0.4999999999999965028 ) ) ;
#5444=CIRCLE ( 'NONE', #10011, 5.000000000000000000 ) ;
#5447=ORIENTED_EDGE ( 'NONE', *, *, #11534, .F. ) ;
#5449=DIRECTION ( 'NONE',  ( -1.776356839400250465E-15, 0.000000000000000000, 1.000000000000000000 ) ) ;
#5457=CARTESIAN_POINT ( 'NONE',  ( 2.143131898507868248E-15, 127.0000000000000000, 17.50000000000000000 ) ) ;
#5464=CARTESIAN_POINT ( 'NONE',  ( -34.17938886450476588, 77.00000000000000000, 8.633741422215349459 ) ) ;
#5466=CARTESIAN_POINT ( 'NONE',  ( -29.05832229253449128, 87.09380371750548022, -8.606096436291647223 ) ) ;
#5470=VERTEX_POINT ( 'NONE', #9524 ) ;
#5488=EDGE_CURVE ( 'NONE', #7769, #1834, #4231, .T. ) ;
#5498=CARTESIAN_POINT ( 'NONE',  ( -30.99900678938364251, 76.83479030960515388, 8.564870178622241426 ) ) ;
#5499=ORIENTED_EDGE ( 'NONE', *, *, #248, .T. ) ;
#5507=VERTEX_POINT ( 'NONE', #5119 ) ;
#5520=EDGE_CURVE ( 'NONE', #6241, #3797, #1169, .T. ) ;
#5522=CARTESIAN_POINT ( 'NONE',  ( 34.84121487603211875, 75.26794919243111792, -7.660254037844449471 ) ) ;
#5530=CARTESIAN_POINT ( 'NONE',  ( -30.43737458073258040, 77.00000000000001421, 5.702507482421638407 ) ) ;
#5532=CARTESIAN_POINT ( 'NONE',  ( -27.32044479829590244, 86.95653975047672191, -12.39329872843003066 ) ) ;
#5541=AXIS2_PLACEMENT_3D ( 'NONE', #3676, #7482, #11294 ) ;
#5552=AXIS2_PLACEMENT_3D ( 'NONE', #4456, #9936, #7205 ) ;
#5556=DIRECTION ( 'NONE',  ( 0.000000000000000000, 1.000000000000000000, 0.000000000000000000 ) ) ;
#5569=CIRCLE ( 'NONE', #1409, 24.99999999999999645 ) ;
#5574=EDGE_LOOP ( 'NONE', ( #331, #8186, #4655, #11529 ) ) ;
#5576=DIRECTION ( 'NONE',  ( 0.000000000000000000, 0.000000000000000000, -1.000000000000000000 ) ) ;
#5583=ORIENTED_EDGE ( 'NONE', *, *, #973, .F. ) ;
#5584=SHAPE_REPRESENTATION_RELATIONSHIP ( 'NONE' , 'NONE' ,  #11842, #4372 ) ;
#5589=CARTESIAN_POINT ( 'NONE',  ( -30.07733313487553772, 77.00000000000709122, 4.660254037819535178 ) ) ;
#5590=CARTESIAN_POINT ( 'NONE',  ( 0.000000000000000000, 92.00000000000000000, 0.000000000000000000 ) ) ;
#5597=EDGE_CURVE ( 'NONE', #5761, #7558, #5237, .T. ) ;
#5603=AXIS2_PLACEMENT_3D ( 'NONE', #4903, #11514, #9807 ) ;
#5606=CARTESIAN_POINT ( 'NONE',  ( 0.000000000000000000, 87.50000000000000000, 0.000000000000000000 ) ) ;
#5614=AXIS2_PLACEMENT_3D ( 'NONE', #7370, #2627, #181 ) ;
#5615=ORIENTED_EDGE ( 'NONE', *, *, #1330, .F. ) ;
#5625=DIRECTION ( 'NONE',  ( 0.000000000000000000, 0.000000000000000000, -1.000000000000000000 ) ) ;
#5627=ORIENTED_EDGE ( 'NONE', *, *, #12180, .T. ) ;
#5629=CARTESIAN_POINT ( 'NONE',  ( 30.00100000000000122, 87.00000000000000000, -8.660254037844435260 ) ) ;
#5631=EDGE_CURVE ( 'NONE', #10799, #7703, #1091, .T. ) ;
#5632=ORIENTED_EDGE ( 'NONE', *, *, #11582, .T. ) ;
#5646=EDGE_CURVE ( 'NONE', #9969, #1793, #4477, .T. ) ;
#5648=AXIS2_PLACEMENT_3D ( 'NONE', #4473, #12092, #3543 ) ;
#5651=ORIENTED_EDGE ( 'NONE', *, *, #2974, .T. ) ;
#5657=AXIS2_PLACEMENT_3D ( 'NONE', #6959, #2222, #6028 ) ;
#5659=UNCERTAINTY_MEASURE_WITH_UNIT (LENGTH_MEASURE( 1.000000000000000082E-05 ), #9241, 'distance_accuracy_value', 'NONE');
#5674=ORIENTED_EDGE ( 'NONE', *, *, #897, .T. ) ;
#5683=LINE ( 'NONE', #12293, #1273 ) ;
#5696=CLOSED_SHELL ( 'NONE', ( #9838, #7689, #8010, #12344, #3651, #6862, #9563, #1558, #8826, #7242, #4236, #4494, #12016, #11381, #10505, #5755, #747, #11597, #3485, #7167, #10541, #683, #1667, #10611, #2830, #2632, #5165, #10739, #12074, #10271, #6602, #6636, #6518, #9491, #4966, #9465, #6760, #7938, #7182, #293, #1607, #224, #9073, #2412, #3227, #6968, #8212, #3991, #4866, #4789, #2915, #11313 ) ) ;
#5705=CIRCLE ( 'NONE', #6099, 17.50000000000000000 ) ;
#5717=CARTESIAN_POINT ( 'NONE',  ( -31.11163258972580081, 76.09530646335886672, 6.227229208586041231 ) ) ;
#5719=EDGE_CURVE ( 'NONE', #10079, #6241, #2775, .T. ) ;
#5720=EDGE_CURVE ( 'NONE', #11439, #10304, #2277, .T. ) ;
#5746=LINE ( 'NONE', #6737, #9373 ) ;
#5755=ADVANCED_FACE ( 'NONE', ( #7351, #1739 ), #4538, .T. ) ;
#5758=ORIENTED_EDGE ( 'NONE', *, *, #10921, .T. ) ;
#5759=CARTESIAN_POINT ( 'NONE',  ( 32.15778161310143446, 87.00000000000000000, 8.660254037844435260 ) ) ;
#5760=LINE ( 'NONE', #4003, #8662 ) ;
#5761=VERTEX_POINT ( 'NONE', #10640 ) ;
#5770=EDGE_LOOP ( 'NONE', ( #9149, #3394, #7807, #8336 ) ) ;
#5791=CIRCLE ( 'NONE', #2771, 17.50000000000000000 ) ;
#5801=CARTESIAN_POINT ( 'NONE',  ( 0.000000000000000000, 122.0000000000000000, -17.50000000000000000 ) ) ;
#5812=AXIS2_PLACEMENT_3D ( 'NONE', #8529, #9525, #5625 ) ;
#5819=EDGE_LOOP ( 'NONE', ( #5033, #4130, #4981, #11855 ) ) ;
#5837=CARTESIAN_POINT ( 'NONE',  ( -69.85388127645425982, 77.00000000000000000, 8.660254037844445918 ) ) ;
#5838=CARTESIAN_POINT ( 'NONE',  ( -30.94187416189151918, 76.19472969970551901, 6.055023111780714729 ) ) ;
#5861=CARTESIAN_POINT ( 'NONE',  ( 32.61619934561887391, 76.99999999999998579, -8.120688671832020589 ) ) ;
#5864=EDGE_CURVE ( 'NONE', #4364, #80, #11578, .T. ) ;
#5866=DIRECTION ( 'NONE',  ( -0.000000000000000000, -1.000000000000000000, -0.000000000000000000 ) ) ;
#5869=( BOUNDED_CURVE ( )  B_SPLINE_CURVE ( 3, ( #6937, #12049, #9092, #7309 ),
 .UNSPECIFIED., .F., .T. ) 
 B_SPLINE_CURVE_WITH_KNOTS ( ( 4, 4 ),
 ( 1.143370257677567281, 1.145717000886475656 ),
 .UNSPECIFIED. ) 
 CURVE ( )  GEOMETRIC_REPRESENTATION_ITEM ( )  RATIONAL_B_SPLINE_CURVE ( ( 1.000000000000000000, 0.9999995410664119788, 0.9999995410664119788, 1.000000000000000000 ) ) 
 REPRESENTATION_ITEM ( '' )  );
#5915=FACE_OUTER_BOUND ( 'NONE', #5819, .T. ) ;
#5919=CARTESIAN_POINT ( 'NONE',  ( -28.20745110743096262, 86.12135132227002998, -11.13838988601301239 ) ) ;
#5930=FACE_OUTER_BOUND ( 'NONE', #724, .T. ) ;
#5939=CIRCLE ( 'NONE', #2344, 15.00000000000000000 ) ;
#5955=VERTEX_POINT ( 'NONE', #8821 ) ;
#5961=ORIENTED_EDGE ( 'NONE', *, *, #5631, .T. ) ;
#5966=CARTESIAN_POINT ( 'NONE',  ( -27.65180490099799115, 87.90152798314358051, -11.49631016393330540 ) ) ;
#5974=VERTEX_POINT ( 'NONE', #4220 ) ;
#5977=EDGE_CURVE ( 'NONE', #8953, #7634, #10009, .T. ) ;
#5979=B_SPLINE_CURVE_WITH_KNOTS ( 'NONE', 3,
 ( #5338, #1659, #5464, #8436, #7457, #8314, #12138, #2649, #1538, #6459, #852, #4394, #1778, #1723, #5530, #12201, #9308, #5589 ),
 .UNSPECIFIED., .F., .F.,
 ( 4, 2, 2, 2, 2, 2, 2, 2, 4 ),
 ( 2.823925224926892107E-17, 0.0008221565609605404907, 0.001644313121921052792, 0.002466469682881565310, 0.003288626243842077395, 0.004110782804802590347, 0.004932939365763108937, 0.005755095926723627527, 0.006577252487684147851 ),
 .UNSPECIFIED. ) ;
#5985=CARTESIAN_POINT ( 'NONE',  ( 27.97213591028574342, 86.27509468223338729, 11.40681812415363972 ) ) ;
#5989=VERTEX_POINT ( 'NONE', #1294 ) ;
#6028=DIRECTION ( 'NONE',  ( 0.000000000000000000, 0.000000000000000000, 1.000000000000000000 ) ) ;
#6029=CARTESIAN_POINT ( 'NONE',  ( -13.00000000000000178, 127.0000000000000000, 7.483314773547879106 ) ) ;
#6035=AXIS2_PLACEMENT_3D ( 'NONE', #12165, #5556, #3677 ) ;
#6036=ORIENTED_EDGE ( 'NONE', *, *, #4290, .F. ) ;
#6042=CARTESIAN_POINT ( 'NONE',  ( 32.13993895771327658, 87.28197645339800204, 8.497454856569966353 ) ) ;
#6045=CARTESIAN_POINT ( 'NONE',  ( 27.54203853141984126, 86.50063778822033100, 11.90690952824018467 ) ) ;
#6053=ORIENTED_EDGE ( 'NONE', *, *, #3515, .F. ) ;
#6067=AXIS2_PLACEMENT_3D ( 'NONE', #12152, #3544, #4346 ) ;
#6099=AXIS2_PLACEMENT_3D ( 'NONE', #4511, #6383, #5576 ) ;
#6101=DIRECTION ( 'NONE',  ( 0.000000000000000000, 1.000000000000000000, 0.000000000000000000 ) ) ;
#6110=ORIENTED_EDGE ( 'NONE', *, *, #9437, .T. ) ;
#6116=CARTESIAN_POINT ( 'NONE',  ( -30.00100000000000122, 77.00000000000000000, -8.660254037844445918 ) ) ;
#6130=ORIENTED_EDGE ( 'NONE', *, *, #11534, .T. ) ;
#6147=CARTESIAN_POINT ( 'NONE',  ( -28.48065962374905169, 85.97961707684488886, -10.89289897176423061 ) ) ;
#6148=CARTESIAN_POINT ( 'NONE',  ( 29.75437749274565391, 83.76094350395922561, 7.050043618115805266 ) ) ;
#6163=ORIENTED_EDGE ( 'NONE', *, *, #11690, .F. ) ;
#6169=EDGE_CURVE ( 'NONE', #6660, #8670, #4677, .T. ) ;
#6208=ORIENTED_EDGE ( 'NONE', *, *, #6710, .F. ) ;
#6216=DIRECTION ( 'NONE',  ( 0.000000000000000000, -0.4999999999999976685, 0.8660254037844399289 ) ) ;
#6237=ORIENTED_EDGE ( 'NONE', *, *, #7617, .T. ) ;
#6241=VERTEX_POINT ( 'NONE', #8110 ) ;
#6247=FACE_OUTER_BOUND ( 'NONE', #6487, .T. ) ;
#6248=DIRECTION ( 'NONE',  ( 0.000000000000000000, 0.000000000000000000, -1.000000000000000000 ) ) ;
#6259=ORIENTED_EDGE ( 'NONE', *, *, #1454, .F. ) ;
#6265=AXIS2_PLACEMENT_3D ( 'NONE', #6657, #6780, #7716 ) ;
#6272=AXIS2_PLACEMENT_3D ( 'NONE', #5606, #6348, #1736 ) ;
#6274=CARTESIAN_POINT ( 'NONE',  ( -27.53586651884020498, 87.45908356336337874, -11.91741659355894889 ) ) ;
#6287=CARTESIAN_POINT ( 'NONE',  ( 31.88521078284830423, 84.50000000000000000, 10.10362971081847228 ) ) ;
#6288=ORIENTED_EDGE ( 'NONE', *, *, #671, .F. ) ;
#6289=FACE_OUTER_BOUND ( 'NONE', #5174, .T. ) ;
#6299=EDGE_CURVE ( 'NONE', #3797, #7113, #7857, .T. ) ;
#6305=CARTESIAN_POINT ( 'NONE',  ( -30.08147999331295352, 76.80445198238156479, 4.520396356853239261 ) ) ;
#6308=DIRECTION ( 'NONE',  ( 0.000000000000000000, -0.8660254037844402619, 0.4999999999999975575 ) ) ;
#6313=CARTESIAN_POINT ( 'NONE',  ( 27.33018067101282966, 87.00000000000000000, 12.37179148263486539 ) ) ;
#6315=EDGE_CURVE ( 'NONE', #8, #8579, #11815, .T. ) ;
#6319=CARTESIAN_POINT ( 'NONE',  ( 0.000000000000000000, 122.5000000000000000, 0.000000000000000000 ) ) ;
#6335=CARTESIAN_POINT ( 'NONE',  ( -27.30089691780743877, 86.86968904112121947, -12.43627868308088935 ) ) ;
#6348=DIRECTION ( 'NONE',  ( 0.000000000000000000, 1.000000000000000000, 0.000000000000000000 ) ) ;
#6352=CARTESIAN_POINT ( 'NONE',  ( 27.46866764507870684, 86.65804127256188849, 12.06796414783009297 ) ) ;
#6358=ORIENTED_EDGE ( 'NONE', *, *, #6627, .F. ) ;
#6366=CARTESIAN_POINT ( 'NONE',  ( -34.80906958247980754, 75.85155757747834571, 7.997200496052795593 ) ) ;
#6369=DIRECTION ( 'NONE',  ( -0.000000000000000000, -1.000000000000000000, -0.000000000000000000 ) ) ;
#6383=DIRECTION ( 'NONE',  ( -0.000000000000000000, -1.000000000000000000, -0.000000000000000000 ) ) ;
#6406=DIRECTION ( 'NONE',  ( 0.000000000000000000, -0.4999999999999976685, -0.8660254037844399289 ) ) ;
#6454=AXIS2_PLACEMENT_3D ( 'NONE', #4616, #3503, #7308 ) ;
#6455=EDGE_CURVE ( 'NONE', #4062, #7098, #188, .T. ) ;
#6456=CARTESIAN_POINT ( 'NONE',  ( 0.000000000000000000, 170.0000000000000000, 0.000000000000000000 ) ) ;
#6459=CARTESIAN_POINT ( 'NONE',  ( -31.52024609858349180, 77.00000000000001421, 7.288261850756687643 ) ) ;
#6464=AXIS2_PLACEMENT_3D ( 'NONE', #373, #4124, #6989 ) ;
#6487=EDGE_LOOP ( 'NONE', ( #5447, #2294, #151, #12318 ) ) ;
#6488=DIRECTION ( 'NONE',  ( 1.224646799147349509E-16, 0.000000000000000000, -1.000000000000000000 ) ) ;
#6489=DIRECTION ( 'NONE',  ( 0.000000000000000000, 0.000000000000000000, 1.000000000000000000 ) ) ;
#6493=DIRECTION ( 'NONE',  ( 0.000000000000000000, 0.4999999999999965028, -0.8660254037844407060 ) ) ;
#6494=CARTESIAN_POINT ( 'NONE',  ( -28.47250777504872943, 87.47929846073044757, -9.490423323819145551 ) ) ;
#6496=CARTESIAN_POINT ( 'NONE',  ( -27.67899820261485999, 88.38261385519929547, -11.05501148229834030 ) ) ;
#6498=CARTESIAN_POINT ( 'NONE',  ( -30.00100000000000122, 85.26794919243110371, 9.660254037844429931 ) ) ;
#6504=CIRCLE ( 'NONE', #4505, 40.00000000000000000 ) ;
#6514=CARTESIAN_POINT ( 'NONE',  ( 0.000000000000000000, 77.00000000000000000, -25.50000000000000000 ) ) ;
#6518=ADVANCED_FACE ( 'NONE', ( #7171 ), #3090, .F. ) ;
#6535=DIRECTION ( 'NONE',  ( -0.000000000000000000, -1.000000000000000000, -0.000000000000000000 ) ) ;
#6538=CARTESIAN_POINT ( 'NONE',  ( 27.69110892066590779, 86.46107124639162578, 11.72680205493499628 ) ) ;
#6542=DIRECTION ( 'NONE',  ( -1.000000000000000000, 0.000000000000000000, 0.000000000000000000 ) ) ;
#6545=DIRECTION ( 'NONE',  ( 0.000000000000000000, 1.000000000000000000, 0.000000000000000000 ) ) ;
#6546=DIRECTION ( 'NONE',  ( 0.000000000000000000, 1.000000000000000000, 0.000000000000000000 ) ) ;
#6553=CARTESIAN_POINT ( 'NONE',  ( -30.00100000000000122, 77.00000000000000000, -8.660254037844445918 ) ) ;
#6583=ORIENTED_EDGE ( 'NONE', *, *, #5646, .T. ) ;
#6602=ADVANCED_FACE ( 'NONE', ( #4358, #7235 ), #11800, .F. ) ;
#6606=DIRECTION ( 'NONE',  ( 0.000000000000000000, -0.8660254037844401509, 0.4999999999999974465 ) ) ;
#6609=CARTESIAN_POINT ( 'NONE',  ( 34.17938886450476588, 77.00000000000000000, -8.633741422215349459 ) ) ;
#6627=EDGE_CURVE ( 'NONE', #6899, #2508, #2841, .T. ) ;
#6630=AXIS2_PLACEMENT_3D ( 'NONE', #11845, #8142, #4226 ) ;
#6633=ORIENTED_EDGE ( 'NONE', *, *, #3640, .T. ) ;
#6636=ADVANCED_FACE ( 'NONE', ( #9459 ), #3048, .F. ) ;
#6637=ORIENTED_EDGE ( 'NONE', *, *, #4016, .T. ) ;
#6653=VECTOR ( 'NONE', #1677, 1000.000000000000000 ) ;
#6654=CARTESIAN_POINT ( 'NONE',  ( -34.84121487603211875, 75.26794919243111792, 7.660254037844449471 ) ) ;
#6657=CARTESIAN_POINT ( 'NONE',  ( 0.000000000000000000, 92.00000000000000000, 0.000000000000000000 ) ) ;
#6660=VERTEX_POINT ( 'NONE', #2616 ) ;
#6676=EDGE_CURVE ( 'NONE', #3231, #2119, #5444, .T. ) ;
#6691=EDGE_LOOP ( 'NONE', ( #1761, #4157, #2453, #2487, #10628, #8114 ) ) ;
#6693=PLANE ( 'NONE',  #5398 ) ;
#6700=AXIS2_PLACEMENT_3D ( 'NONE', #10874, #3335, #11698 ) ;
#6703=CARTESIAN_POINT ( 'NONE',  ( 0.000000000000000000, 122.0000000000000000, 0.000000000000000000 ) ) ;
#6705=FACE_OUTER_BOUND ( 'NONE', #2089, .T. ) ;
#6706=CARTESIAN_POINT ( 'NONE',  ( 45.35898384862240107, 86.99999999999997158, 8.660254037844424602 ) ) ;
#6710=EDGE_CURVE ( 'NONE', #9853, #3368, #11002, .T. ) ;
#6715=FACE_OUTER_BOUND ( 'NONE', #10568, .T. ) ;
#6723=CARTESIAN_POINT ( 'NONE',  ( 0.000000000000000000, 216.0365690573663926, 0.000000000000000000 ) ) ;
#6726=EDGE_CURVE ( 'NONE', #6910, #5955, #10277, .T. ) ;
#6728=DIRECTION ( 'NONE',  ( 0.000000000000000000, 0.000000000000000000, -1.000000000000000000 ) ) ;
#6737=CARTESIAN_POINT ( 'NONE',  ( 30.00100000000000122, 77.00000000000000000, 4.660254037844413944 ) ) ;
#6760=ADVANCED_FACE ( 'NONE', ( #2800 ), #8523, .T. ) ;
#6769=APPLICATION_CONTEXT ( 'automotive_design' ) ;
#6778=ORIENTED_EDGE ( 'NONE', *, *, #6726, .T. ) ;
#6780=DIRECTION ( 'NONE',  ( 0.000000000000000000, 1.000000000000000000, 0.000000000000000000 ) ) ;
#6781=VECTOR ( 'NONE', #2963, 1000.000000000000000 ) ;
#6794=CARTESIAN_POINT ( 'NONE',  ( 34.73110591274434000, 77.00000000000000000, -8.660254037844445918 ) ) ;
#6810=ORIENTED_EDGE ( 'NONE', *, *, #8299, .F. ) ;
#6816=CARTESIAN_POINT ( 'NONE',  ( 0.000000000000000000, 122.0000000000000000, 17.00000000000000000 ) ) ;
#6827=DIRECTION ( 'NONE',  ( 8.881784197001252323E-16, 0.000000000000000000, 1.000000000000000000 ) ) ;
#6832=EDGE_LOOP ( 'NONE', ( #4987, #4858 ) ) ;
#6835=CIRCLE ( 'NONE', #1069, 24.99999999999999645 ) ;
#6839=DIRECTION ( 'NONE',  ( 0.000000000000000000, 0.000000000000000000, 1.000000000000000000 ) ) ;
#6840=ORIENTED_EDGE ( 'NONE', *, *, #2975, .T. ) ;
#6841=DIRECTION ( 'NONE',  ( 1.000000000000000000, 0.000000000000000000, 0.000000000000000000 ) ) ;
#6844=CARTESIAN_POINT ( 'NONE',  ( -32.15778161310143446, 87.00000000000000000, -8.660254037844435260 ) ) ;
#6846=ORIENTED_EDGE ( 'NONE', *, *, #11505, .T. ) ;
#6854=FACE_OUTER_BOUND ( 'NONE', #5425, .T. ) ;
#6862=ADVANCED_FACE ( 'NONE', ( #6854 ), #8831, .F. ) ;
#6876=DIRECTION ( 'NONE',  ( -0.000000000000000000, -1.000000000000000000, -0.000000000000000000 ) ) ;
#6882=AXIS2_PLACEMENT_3D ( 'NONE', #734, #4528, #12141 ) ;
#6899=VERTEX_POINT ( 'NONE', #4408 ) ;
#6910=VERTEX_POINT ( 'NONE', #2483 ) ;
#6917=DIRECTION ( 'NONE',  ( -0.000000000000000000, -1.000000000000000000, -0.000000000000000000 ) ) ;
#6927=EDGE_CURVE ( 'NONE', #10169, #11869, #2645, .T. ) ;
#6928=FACE_OUTER_BOUND ( 'NONE', #5018, .T. ) ;
#6930=EDGE_CURVE ( 'NONE', #10079, #3797, #4234, .T. ) ;
#6937=CARTESIAN_POINT ( 'NONE',  ( -27.30107202361637775, 86.87046582918780757, -12.43589427268144831 ) ) ;
#6939=ORIENTED_EDGE ( 'NONE', *, *, #8037, .F. ) ;
#6944=ORIENTED_EDGE ( 'NONE', *, *, #8620, .T. ) ;
#6946=ORIENTED_EDGE ( 'NONE', *, *, #5259, .T. ) ;
#6956=AXIS2_PLACEMENT_3D ( 'NONE', #7279, #9124, #4825 ) ;
#6959=CARTESIAN_POINT ( 'NONE',  ( 0.000000000000000000, 87.00000000000000000, 24.99999999999999645 ) ) ;
#6968=ADVANCED_FACE ( 'NONE', ( #10773 ), #2041, .F. ) ;
#6971=CIRCLE ( 'NONE', #9551, 40.00000000000000000 ) ;
#6977=CARTESIAN_POINT ( 'NONE',  ( -45.35898384862240107, 85.26794919243110371, -9.660254037844429931 ) ) ;
#6979=ORIENTED_EDGE ( 'NONE', *, *, #9336, .F. ) ;
#6981=CIRCLE ( 'NONE', #4790, 5.000000000000000888 ) ;
#6984=EDGE_CURVE ( 'NONE', #7967, #3932, #6835, .T. ) ;
#6986=CARTESIAN_POINT ( 'NONE',  ( 28.61611180472260330, 87.72948999988453522, 9.923767781257849308 ) ) ;
#6988=ORIENTED_EDGE ( 'NONE', *, *, #6627, .T. ) ;
#6989=DIRECTION ( 'NONE',  ( 0.000000000000000000, 0.000000000000000000, 1.000000000000000000 ) ) ;
#6991=AXIS2_PLACEMENT_3D ( 'NONE', #5137, #380, #6248 ) ;
#6998=AXIS2_PLACEMENT_3D ( 'NONE', #7768, #1689, #1044 ) ;
#7018=VERTEX_POINT ( 'NONE', #928 ) ;
#7035=LINE ( 'NONE', #425, #7489 ) ;
#7036=ORIENTED_EDGE ( 'NONE', *, *, #7330, .T. ) ;
#7038=( BOUNDED_SURFACE ( )  B_SPLINE_SURFACE ( 3, 2, ( 
 ( #6305, #10089, #1690 ),
 ( #12109, #11298, #6366 ),
 ( #7428, #820, #2559 ),
 ( #11230, #5498, #759 ) ),
 .UNSPECIFIED., .F., .F., .F. ) 
 B_SPLINE_SURFACE_WITH_KNOTS ( ( 4, 4 ),
 ( 3, 3 ),
 ( 1.665911834627059607, 1.695449464845517618 ),
 ( 0.2468956587999593388, 1.000000000000000000 ),
 .UNSPECIFIED. ) 
 GEOMETRIC_REPRESENTATION_ITEM ( )  RATIONAL_B_SPLINE_SURFACE ( (
 ( 0.8800340755151767613, 0.7570513692546891882, 1.000000000000000000),
 ( 0.8788691223080344894, 0.7546921677749939272, 1.000000000000000000),
 ( 0.8776977286441711712, 0.7523199234237630817, 1.000000000000000000),
 ( 0.8765201392483088494, 0.7499351318045301973, 1.000000000000000000) ) ) 
 REPRESENTATION_ITEM ( '' )  SURFACE ( )  );
#7043=CIRCLE ( 'NONE', #10822, 15.00000000000000000 ) ;
#7045=ORIENTED_EDGE ( 'NONE', *, *, #10672, .F. ) ;
#7050=DIRECTION ( 'NONE',  ( 0.000000000000000000, 0.000000000000000000, 1.000000000000000000 ) ) ;
#7054=AXIS2_PLACEMENT_3D ( 'NONE', #7620, #11249, #10296 ) ;
#7077=CIRCLE ( 'NONE', #6454, 25.50000000000000000 ) ;
#7080=VERTEX_POINT ( 'NONE', #10199 ) ;
#7087=AXIS2_PLACEMENT_3D ( 'NONE', #11940, #2523, #944 ) ;
#7089=CARTESIAN_POINT ( 'NONE',  ( 31.48070082314331231, 75.91043305631261262, -6.547439342558601716 ) ) ;
#7096=ORIENTED_EDGE ( 'NONE', *, *, #2085, .T. ) ;
#7097=CARTESIAN_POINT ( 'NONE',  ( 32.21610632498789073, 86.34645847305445443, 9.037576414353038601 ) ) ;
#7098=VERTEX_POINT ( 'NONE', #7411 ) ;
#7101=VERTEX_POINT ( 'NONE', #12212 ) ;
#7110=CARTESIAN_POINT ( 'NONE',  ( 28.14852131675075597, 87.98519278820045031, 10.36665800225805611 ) ) ;
#7112=DIRECTION ( 'NONE',  ( 0.000000000000000000, 1.000000000000000000, 0.000000000000000000 ) ) ;
#7113=VERTEX_POINT ( 'NONE', #10320 ) ;
#7116=ORIENTED_EDGE ( 'NONE', *, *, #3609, .F. ) ;
#7119=CARTESIAN_POINT ( 'NONE',  ( 1.836970198721029589E-15, 170.0000000000000000, 15.00000000000000000 ) ) ;
#7130=ORIENTED_EDGE ( 'NONE', *, *, #10921, .F. ) ;
#7140=LINE ( 'NONE', #10059, #1872 ) ;
#7147=CARTESIAN_POINT ( 'NONE',  ( 31.11163258972580081, 76.09530646335886672, -6.227229208586041231 ) ) ;
#7167=ADVANCED_FACE ( 'NONE', ( #9196 ), #674, .T. ) ;
#7171=FACE_OUTER_BOUND ( 'NONE', #1885, .T. ) ;
#7179=FACE_OUTER_BOUND ( 'NONE', #5574, .T. ) ;
#7182=ADVANCED_FACE ( 'NONE', ( #6715 ), #11461, .T. ) ;
#7184=AXIS2_PLACEMENT_3D ( 'NONE', #11054, #7318, #9290 ) ;
#7195=FACE_OUTER_BOUND ( 'NONE', #142, .T. ) ;
#7205=DIRECTION ( 'NONE',  ( 0.000000000000000000, 0.4999999999999962808, -0.8660254037844407060 ) ) ;
#7209=CARTESIAN_POINT ( 'NONE',  ( 45.35898384862240107, 85.26794919243110371, 9.660254037844419273 ) ) ;
#7211=DIRECTION ( 'NONE',  ( -0.000000000000000000, 1.000000000000000000, -0.000000000000000000 ) ) ;
#7224=VERTEX_POINT ( 'NONE', #9627 ) ;
#7227=CARTESIAN_POINT ( 'NONE',  ( -31.92482683647865471, 87.00000000000005684, -8.660254037844584474 ) ) ;
#7229=EDGE_CURVE ( 'NONE', #8, #10079, #4640, .T. ) ;
#7234=CARTESIAN_POINT ( 'NONE',  ( 29.99337288235791732, 77.98292469156852746, -5.126776908431767588 ) ) ;
#7235=FACE_OUTER_BOUND ( 'NONE', #2519, .T. ) ;
#7236=VERTEX_POINT ( 'NONE', #3035 ) ;
#7242=ADVANCED_FACE ( 'NONE', ( #4033 ), #7828, .T. ) ;
#7246=CIRCLE ( 'NONE', #12024, 5.000000000000000888 ) ;
#7248=DIRECTION ( 'NONE',  ( -0.000000000000000000, -1.000000000000000000, -0.000000000000000000 ) ) ;
#7263=ORIENTED_EDGE ( 'NONE', *, *, #2183, .F. ) ;
#7268=PLANE ( 'NONE',  #68 ) ;
#7275=CARTESIAN_POINT ( 'NONE',  ( -27.33018067101281900, 86.99999999999998579, -12.37179148263487782 ) ) ;
#7279=CARTESIAN_POINT ( 'NONE',  ( 0.000000000000000000, 170.0000000000000000, 0.000000000000000000 ) ) ;
#7280=DIRECTION ( 'NONE',  ( -0.000000000000000000, 0.8660254037844402619, -0.4999999999999975575 ) ) ;
#7284=CIRCLE ( 'NONE', #1719, 24.99999999999999645 ) ;
#7289=DIRECTION ( 'NONE',  ( -0.000000000000000000, -1.000000000000000000, -0.000000000000000000 ) ) ;
#7295=CARTESIAN_POINT ( 'NONE',  ( 0.000000000000000000, 87.00000000000000000, 24.99999999999999645 ) ) ;
#7301=DIRECTION ( 'NONE',  ( 0.000000000000000000, 0.000000000000000000, 1.000000000000000000 ) ) ;
#7308=DIRECTION ( 'NONE',  ( 0.000000000000000000, 0.000000000000000000, -1.000000000000000000 ) ) ;
#7309=CARTESIAN_POINT ( 'NONE',  ( -27.33018067101282256, 87.00000000000000000, -12.37179148263487605 ) ) ;
#7318=DIRECTION ( 'NONE',  ( 0.000000000000000000, -0.8660254037844401509, -0.4999999999999974465 ) ) ;
#7324=CARTESIAN_POINT ( 'NONE',  ( -30.43816488677641985, 80.28464834591375165, 2.971076217724743618 ) ) ;
#7325=CARTESIAN_POINT ( 'NONE',  ( -27.33018067101282256, 87.00000000000000000, -12.37179148263487605 ) ) ;
#7329=ORIENTED_EDGE ( 'NONE', *, *, #5221, .T. ) ;
#7330=EDGE_CURVE ( 'NONE', #5470, #4117, #2469, .T. ) ;
#7334=DIRECTION ( 'NONE',  ( 0.000000000000000000, -0.4999999999999976685, -0.8660254037844399289 ) ) ;
#7351=FACE_OUTER_BOUND ( 'NONE', #1679, .T. ) ;
#7362=AXIS2_PLACEMENT_3D ( 'NONE', #4748, #3817, #5000 ) ;
#7369=CARTESIAN_POINT ( 'NONE',  ( 0.000000000000000000, 122.0000000000000000, -22.00000000000000355 ) ) ;
#7370=CARTESIAN_POINT ( 'NONE',  ( 0.000000000000000000, 122.5000000000000000, 0.000000000000000000 ) ) ;
#7375=AXIS2_PLACEMENT_3D ( 'NONE', #2856, #6542, #10330 ) ;
#7377=ORIENTED_EDGE ( 'NONE', *, *, #1845, .T. ) ;
#7380=ORIENTED_EDGE ( 'NONE', *, *, #7644, .F. ) ;
#7387=CARTESIAN_POINT ( 'NONE',  ( 0.000000000000000000, 92.00000000000000000, -22.00000000000000355 ) ) ;
#7399=CARTESIAN_POINT ( 'NONE',  ( -8.500000000000000000, 122.5000000000000000, -6.164414002968973350 ) ) ;
#7400=AXIS2_PLACEMENT_3D ( 'NONE', #2061, #5866, #4805 ) ;
#7411=CARTESIAN_POINT ( 'NONE',  ( 0.000000000000000000, 87.50000000000000000, -17.50000000000000000 ) ) ;
#7412=CARTESIAN_POINT ( 'NONE',  ( -8.500000000000000000, 165.5000000000000000, -6.164414002968973350 ) ) ;
#7428=CARTESIAN_POINT ( 'NONE',  ( -29.99337288235791732, 77.98292469156852746, 5.126776908431767588 ) ) ;
#7432=PLANE ( 'NONE',  #2621 ) ;
#7444=VECTOR ( 'NONE', #2281, 1000.000000000000000 ) ;
#7456=EDGE_CURVE ( 'NONE', #7513, #5974, #7246, .T. ) ;
#7457=CARTESIAN_POINT ( 'NONE',  ( -33.37417589188917333, 76.99999999999998579, 8.451338748825380165 ) ) ;
#7465=EDGE_CURVE ( 'NONE', #6241, #7101, #9746, .T. ) ;
#7477=AXIS2_PLACEMENT_3D ( 'NONE', #9026, #7112, #7301 ) ;
#7478=ORIENTED_EDGE ( 'NONE', *, *, #8506, .F. ) ;
#7480=EDGE_CURVE ( 'NONE', #1112, #7967, #11018, .T. ) ;
#7482=DIRECTION ( 'NONE',  ( 0.000000000000000000, 1.000000000000000000, 0.000000000000000000 ) ) ;
#7484=VERTEX_POINT ( 'NONE', #9814 ) ;
#7489=VECTOR ( 'NONE', #7289, 1000.000000000000000 ) ;
#7499=FACE_OUTER_BOUND ( 'NONE', #8623, .T. ) ;
#7510=ORIENTED_EDGE ( 'NONE', *, *, #1657, .T. ) ;
#7513=VERTEX_POINT ( 'NONE', #8254 ) ;
#7525=VERTEX_POINT ( 'NONE', #4457 ) ;
#7526=CIRCLE ( 'NONE', #5541, 17.50000000000000000 ) ;
#7531=CARTESIAN_POINT ( 'NONE',  ( 2.694222958124177204E-15, 127.0000000000000000, 22.00000000000000355 ) ) ;
#7532=CARTESIAN_POINT ( 'NONE',  ( 0.000000000000000000, 77.00000000000000000, -30.00000000000000000 ) ) ;
#7538=( BOUNDED_SURFACE ( )  B_SPLINE_SURFACE ( 3, 2, ( 
 ( #4584, #10251, #7275 ),
 ( #2534, #1600, #5532 ),
 ( #10064, #9311, #9121 ),
 ( #11201, #3652, #6335 ) ),
 .UNSPECIFIED., .F., .F., .F. ) 
 B_SPLINE_SURFACE_WITH_KNOTS ( ( 4, 4 ),
 ( 3, 3 ),
 ( 5.137468306293111020, 5.139829129961272614 ),
 ( 0.7666061298070812047, 1.000000000000000000 ),
 .UNSPECIFIED. ) 
 GEOMETRIC_REPRESENTATION_ITEM ( )  RATIONAL_B_SPLINE_SURFACE ( (
 ( 0.9369318869591372057, 0.9588653738936746551, 1.000000000000000000),
 ( 0.9369993130727753972, 0.9589093509185225850, 1.000000000000000000),
 ( 0.9370666800230464943, 0.9589532893555189341, 1.000000000000000000),
 ( 0.9371339877439295307, 0.9589971891616031474, 1.000000000000000000) ) ) 
 REPRESENTATION_ITEM ( '' )  SURFACE ( )  );
#7541=DIRECTION ( 'NONE',  ( -5.551115123125782702E-15, -0.4999999999999976685, 0.8660254037844399289 ) ) ;
#7542=ORIENTED_EDGE ( 'NONE', *, *, #10146, .T. ) ;
#7552=PLANE ( 'NONE',  #5006 ) ;
#7558=VERTEX_POINT ( 'NONE', #661 ) ;
#7560=CARTESIAN_POINT ( 'NONE',  ( 0.000000000000000000, 216.0365690573663926, 0.000000000000000000 ) ) ;
#7573=CARTESIAN_POINT ( 'NONE',  ( 0.000000000000000000, 165.5000000000000000, -10.49999999999999822 ) ) ;
#7596=AXIS2_PLACEMENT_3D ( 'NONE', #6553, #2742, #1939 ) ;
#7597=EDGE_CURVE ( 'NONE', #12062, #12288, #5979, .T. ) ;
#7602=CARTESIAN_POINT ( 'NONE',  ( 31.52024609858349180, 77.00000000000001421, -7.288261850756687643 ) ) ;
#7608=PLANE ( 'NONE',  #7596 ) ;
#7610=( BOUNDED_CURVE ( )  B_SPLINE_CURVE ( 3, ( #3134, #9851, #1448, #506 ),
 .UNSPECIFIED., .F., .F. ) 
 B_SPLINE_CURVE_WITH_KNOTS ( ( 4, 4 ),
 ( 4.284962911267360397, 4.868362425771961099 ),
 .UNSPECIFIED. ) 
 CURVE ( )  GEOMETRIC_REPRESENTATION_ITEM ( )  RATIONAL_B_SPLINE_CURVE ( ( 1.000000000000000000, 0.9718376280744367435, 0.9718376280744367435, 1.000000000000000000 ) ) 
 REPRESENTATION_ITEM ( '' )  );
#7617=EDGE_CURVE ( 'NONE', #80, #5761, #8190, .T. ) ;
#7620=CARTESIAN_POINT ( 'NONE',  ( 0.000000000000000000, 77.00000000000000000, 0.000000000000000000 ) ) ;
#7623=DIRECTION ( 'NONE',  ( 0.000000000000000000, -0.4999999999999965028, 0.8660254037844407060 ) ) ;
#7625=AXIS2_PLACEMENT_3D ( 'NONE', #4729, #6606, #10400 ) ;
#7631=ORIENTED_EDGE ( 'NONE', *, *, #8275, .F. ) ;
#7634=VERTEX_POINT ( 'NONE', #4765 ) ;
#7644=EDGE_CURVE ( 'NONE', #9024, #7513, #8402, .T. ) ;
#7650=CARTESIAN_POINT ( 'NONE',  ( 2.143131898507868248E-15, 122.0000000000000000, 17.50000000000000000 ) ) ;
#7660=CARTESIAN_POINT ( 'NONE',  ( 0.000000000000000000, 127.0000000000000000, 0.000000000000000000 ) ) ;
#7662=CARTESIAN_POINT ( 'NONE',  ( 30.07733313487553772, 77.00000000000709122, -4.660254037819535178 ) ) ;
#7663=CARTESIAN_POINT ( 'NONE',  ( 27.31068353816013783, 86.91310272383458368, 12.41479448187959278 ) ) ;
#7676=PLANE ( 'NONE',  #7362 ) ;
#7683=LINE ( 'NONE', #9723, #1309 ) ;
#7689=ADVANCED_FACE ( 'NONE', ( #6705 ), #10796, .F. ) ;
#7695=FACE_BOUND ( 'NONE', #2669, .T. ) ;
#7696=ORIENTED_EDGE ( 'NONE', *, *, #2019, .F. ) ;
#7697=CARTESIAN_POINT ( 'NONE',  ( 0.000000000000000000, 87.00000000000000000, 0.000000000000000000 ) ) ;
#7698=LINE ( 'NONE', #11512, #6781 ) ;
#7703=VERTEX_POINT ( 'NONE', #3025 ) ;
#7716=DIRECTION ( 'NONE',  ( 0.000000000000000000, -0.000000000000000000, 1.000000000000000000 ) ) ;
#7717=DIRECTION ( 'NONE',  ( -0.000000000000000000, 1.000000000000000000, -0.000000000000000000 ) ) ;
#7720=AXIS2_PLACEMENT_3D ( 'NONE', #1626, #10211, #6488 ) ;
#7725=CARTESIAN_POINT ( 'NONE',  ( 0.000000000000000000, 87.00000000000000000, -25.50000000000000000 ) ) ;
#7728=ORIENTED_EDGE ( 'NONE', *, *, #4389, .F. ) ;
#7747=CARTESIAN_POINT ( 'NONE',  ( -27.46866764507868908, 86.65804127256191691, -12.06796414783013027 ) ) ;
#7751=AXIS2_PLACEMENT_3D ( 'NONE', #10120, #3532, #7334 ) ;
#7768=CARTESIAN_POINT ( 'NONE',  ( 0.000000000000000000, 87.00000000000000000, 0.000000000000000000 ) ) ;
#7769=VERTEX_POINT ( 'NONE', #8806 ) ;
#7772=ORIENTED_EDGE ( 'NONE', *, *, #1760, .T. ) ;
#7792=CARTESIAN_POINT ( 'NONE',  ( 3.245314017740478073E-16, 165.5000000000000000, -2.649999999999993694 ) ) ;
#7799=CIRCLE ( 'NONE', #1630, 5.000000000000000000 ) ;
#7807=ORIENTED_EDGE ( 'NONE', *, *, #8037, .T. ) ;
#7808=CARTESIAN_POINT ( 'NONE',  ( -30.00100000000000122, 87.00000000000000000, 8.660254037844435260 ) ) ;
#7813=AXIS2_PLACEMENT_3D ( 'NONE', #1399, #2330, #5208 ) ;
#7823=DIRECTION ( 'NONE',  ( 0.000000000000000000, 0.000000000000000000, 1.000000000000000000 ) ) ;
#7828=CYLINDRICAL_SURFACE ( 'NONE', #1854, 15.00000000000000000 ) ;
#7829=DIRECTION ( 'NONE',  ( 0.000000000000000000, 1.000000000000000000, 0.000000000000000000 ) ) ;
#7834=FACE_OUTER_BOUND ( 'NONE', #9678, .T. ) ;
#7853=CARTESIAN_POINT ( 'NONE',  ( -8.500000000000000000, 165.5000000000000000, 6.164414002968973350 ) ) ;
#7856=ORIENTED_EDGE ( 'NONE', *, *, #9336, .T. ) ;
#7857=CIRCLE ( 'NONE', #2683, 30.00000000000000000 ) ;
#7873=DIRECTION ( 'NONE',  ( -0.000000000000000000, -1.000000000000000000, -0.000000000000000000 ) ) ;
#7875=EDGE_LOOP ( 'NONE', ( #1436, #4361, #3520, #11445 ) ) ;
#7877=AXIS2_PLACEMENT_3D ( 'NONE', #6703, #144, #1155 ) ;
#7878=CARTESIAN_POINT ( 'NONE',  ( 27.67899820261485999, 88.38261385519929547, 11.05501148229834030 ) ) ;
#7896=ORIENTED_EDGE ( 'NONE', *, *, #2806, .T. ) ;
#7899=CARTESIAN_POINT ( 'NONE',  ( 34.77260134704101802, 76.42358343581042845, -8.327459779344241753 ) ) ;
#7909=CARTESIAN_POINT ( 'NONE',  ( 31.00813199677072873, 87.06416249055504863, 8.771386731425977246 ) ) ;
#7914=CIRCLE ( 'NONE', #3349, 25.50000000000000000 ) ;
#7920=LINE ( 'NONE', #11501, #10566 ) ;
#7921=ORIENTED_EDGE ( 'NONE', *, *, #6984, .F. ) ;
#7938=ADVANCED_FACE ( 'NONE', ( #9867 ), #7993, .T. ) ;
#7961=CARTESIAN_POINT ( 'NONE',  ( 27.30107202361637775, 86.87046582918780757, 12.43589427268144831 ) ) ;
#7967=VERTEX_POINT ( 'NONE', #12002 ) ;
#7984=CIRCLE ( 'NONE', #429, 5.000000000000000888 ) ;
#7993=CYLINDRICAL_SURFACE ( 'NONE', #7813, 40.00000000000000000 ) ;
#7997=ORIENTED_EDGE ( 'NONE', *, *, #4145, .F. ) ;
#8010=ADVANCED_FACE ( 'NONE', ( #718 ), #2304, .F. ) ;
#8016=B_SPLINE_CURVE_WITH_KNOTS ( 'NONE', 3,
 ( #10626, #10563, #2033, #4027, #25, #5838, #5717, #1159, #3840, #2903, #3963, #10440, #11389, #11574 ),
 .UNSPECIFIED., .F., .F.,
 ( 4, 2, 2, 2, 2, 2, 4 ),
 ( 0.001978049138782353184, 0.002761379211137155940, 0.003544709283491958261, 0.004328039355846760583, 0.005111369428201563772, 0.006678029572911168416, 0.008244689717620771324 ),
 .UNSPECIFIED. ) ;
#8034=DIRECTION ( 'NONE',  ( 0.000000000000000000, 1.000000000000000000, 0.000000000000000000 ) ) ;
#8037=EDGE_CURVE ( 'NONE', #1569, #7018, #10063, .T. ) ;
#8044=EDGE_CURVE ( 'NONE', #10772, #5989, #2518, .T. ) ;
#8046=AXIS2_PLACEMENT_3D ( 'NONE', #5296, #8833, #8084 ) ;
#8064=CIRCLE ( 'NONE', #7877, 22.00000000000000355 ) ;
#8076=CARTESIAN_POINT ( 'NONE',  ( -13.00000000000000178, 216.0365690573663926, -7.483314773547880883 ) ) ;
#8084=DIRECTION ( 'NONE',  ( 0.000000000000000000, 0.000000000000000000, 1.000000000000000000 ) ) ;
#8085=CARTESIAN_POINT ( 'NONE',  ( 0.000000000000000000, 92.00000000000000000, 0.000000000000000000 ) ) ;
#8090=ORIENTED_EDGE ( 'NONE', *, *, #11885, .T. ) ;
#8099=ORIENTED_EDGE ( 'NONE', *, *, #2233, .F. ) ;
#8104=CYLINDRICAL_SURFACE ( 'NONE', #9345, 22.00000000000000355 ) ;
#8110=CARTESIAN_POINT ( 'NONE',  ( 27.30107202361637775, 86.87046582918780757, 12.43589427268144831 ) ) ;
#8114=ORIENTED_EDGE ( 'NONE', *, *, #1301, .T. ) ;
#8115=EDGE_CURVE ( 'NONE', #5989, #12062, #11718, .T. ) ;
#8131=CARTESIAN_POINT ( 'NONE',  ( -29.00531465893046601, 86.42397445338744433, -8.992822542244219619 ) ) ;
#8141=EDGE_LOOP ( 'NONE', ( #11092, #12086, #4599 ) ) ;
#8142=DIRECTION ( 'NONE',  ( 0.000000000000000000, 1.000000000000000000, 0.000000000000000000 ) ) ;
#8146=ORIENTED_EDGE ( 'NONE', *, *, #6299, .F. ) ;
#8172=CIRCLE ( 'NONE', #11177, 30.00000000000000000 ) ;
#8186=ORIENTED_EDGE ( 'NONE', *, *, #5977, .T. ) ;
#8189=CARTESIAN_POINT ( 'NONE',  ( -27.96741528345882344, 86.27927944434871677, -11.41192941739715927 ) ) ;
#8190=LINE ( 'NONE', #11449, #11403 ) ;
#8192=CARTESIAN_POINT ( 'NONE',  ( -31.88521078284829713, 84.49999999999997158, -10.10362971081849004 ) ) ;
#8193=CARTESIAN_POINT ( 'NONE',  ( 34.84121487603211875, 75.26794919243111792, -7.660254037844449471 ) ) ;
#8212=ADVANCED_FACE ( 'NONE', ( #11663 ), #10463, .F. ) ;
#8215=ORIENTED_EDGE ( 'NONE', *, *, #10811, .F. ) ;
#8216=CARTESIAN_POINT ( 'NONE',  ( 0.000000000000000000, 122.5000000000000000, 0.000000000000000000 ) ) ;
#8219=PLANE ( 'NONE',  #3813 ) ;
#8251=DIRECTION ( 'NONE',  ( 0.000000000000000000, -0.000000000000000000, 1.000000000000000000 ) ) ;
#8253=CARTESIAN_POINT ( 'NONE',  ( -29.09218482426048524, 85.72793236853334520, -10.45696826948038982 ) ) ;
#8254=CARTESIAN_POINT ( 'NONE',  ( 0.000000000000000000, 87.00000000000000000, -30.00000000000000000 ) ) ;
#8258=CARTESIAN_POINT ( 'NONE',  ( -27.33018067101282256, 86.99999999999998579, -12.37179148263487960 ) ) ;
#8260=DIRECTION ( 'NONE',  ( 0.000000000000000000, 0.000000000000000000, 1.000000000000000000 ) ) ;
#8265=DIRECTION ( 'NONE',  ( 0.000000000000000000, -0.4999999999999976685, 0.8660254037844399289 ) ) ;
#8275=EDGE_CURVE ( 'NONE', #5974, #7236, #7284, .T. ) ;
#8285=CARTESIAN_POINT ( 'NONE',  ( -27.67899820261485999, 88.38261385519929547, -11.05501148229834030 ) ) ;
#8289=DIRECTION ( 'NONE',  ( 0.000000000000000000, 0.000000000000000000, 1.000000000000000000 ) ) ;
#8290=FACE_OUTER_BOUND ( 'NONE', #3737, .T. ) ;
#8299=EDGE_CURVE ( 'NONE', #9853, #6660, #7035, .T. ) ;
#8312=PLANE ( 'NONE',  #5062 ) ;
#8314=CARTESIAN_POINT ( 'NONE',  ( -32.86043907464384972, 76.99999999999998579, 8.246007242324683517 ) ) ;
#8336=ORIENTED_EDGE ( 'NONE', *, *, #638, .F. ) ;
#8348=CARTESIAN_POINT ( 'NONE',  ( 0.000000000000000000, 77.00000000000000000, 0.000000000000000000 ) ) ;
#8392=EDGE_CURVE ( 'NONE', #2119, #3216, #4475, .T. ) ;
#8402=CIRCLE ( 'NONE', #3042, 30.00000000000000000 ) ;
#8413=ORIENTED_EDGE ( 'NONE', *, *, #5597, .T. ) ;
#8416=DIRECTION ( 'NONE',  ( 0.000000000000000000, -0.8660254037844401509, -0.4999999999999974465 ) ) ;
#8421=CARTESIAN_POINT ( 'NONE',  ( 32.05000697088088657, 85.26794919243110371, 9.660254037844429931 ) ) ;
#8424=ORIENTED_EDGE ( 'NONE', *, *, #2844, .F. ) ;
#8436=CARTESIAN_POINT ( 'NONE',  ( -33.64113847583112715, 77.00000000000000000, 8.529771698700599813 ) ) ;
#8441=ORIENTED_EDGE ( 'NONE', *, *, #5719, .F. ) ;
#8458=ORIENTED_EDGE ( 'NONE', *, *, #11354, .T. ) ;
#8491=EDGE_CURVE ( 'NONE', #931, #10229, #1799, .T. ) ;
#8494=( LENGTH_UNIT ( ) NAMED_UNIT ( * ) SI_UNIT ( .MILLI., .METRE. ) );
#8502=ORIENTED_EDGE ( 'NONE', *, *, #5720, .T. ) ;
#8506=EDGE_CURVE ( 'NONE', #7558, #3231, #6504, .T. ) ;
#8523=PLANE ( 'NONE',  #7625 ) ;
#8525=CARTESIAN_POINT ( 'NONE',  ( 31.92904760676809062, 76.99999999999998579, -7.658217335466646070 ) ) ;
#8529=CARTESIAN_POINT ( 'NONE',  ( 0.000000000000000000, 92.00000000000000000, 0.000000000000000000 ) ) ;
#8530=DIRECTION ( 'NONE',  ( 0.000000000000000000, 0.000000000000000000, 1.000000000000000000 ) ) ;
#8537=ORIENTED_EDGE ( 'NONE', *, *, #10811, .T. ) ;
#8547=DIRECTION ( 'NONE',  ( 1.000000000000000000, 0.000000000000000000, 0.000000000000000000 ) ) ;
#8555=VERTEX_POINT ( 'NONE', #11774 ) ;
#8566=B_SPLINE_CURVE_WITH_KNOTS ( 'NONE', 3,
 ( #6313, #771, #640, #2568 ),
 .UNSPECIFIED., .F., .F.,
 ( 4, 4 ),
 ( 0.000000000000000000, 0.001940928724149413795 ),
 .UNSPECIFIED. ) ;
#8577=AXIS2_PLACEMENT_3D ( 'NONE', #10974, #9213, #11802 ) ;
#8579=VERTEX_POINT ( 'NONE', #7209 ) ;
#8586=CARTESIAN_POINT ( 'NONE',  ( 30.55702146375036676, 77.00000000000001421, -5.949569453687718834 ) ) ;
#8611=DIRECTION ( 'NONE',  ( 0.000000000000000000, 0.8660254037844407060, 0.4999999999999965028 ) ) ;
#8618=VERTEX_POINT ( 'NONE', #2593 ) ;
#8620=EDGE_CURVE ( 'NONE', #10587, #7484, #1783, .T. ) ;
#8622=PLANE ( 'NONE',  #10259 ) ;
#8623=EDGE_LOOP ( 'NONE', ( #4927, #8215, #8640, #3613, #7510, #6633, #2724, #2201, #4368 ) ) ;
#8632=CIRCLE ( 'NONE', #6464, 30.00000000000000000 ) ;
#8635=DIRECTION ( 'NONE',  ( 0.000000000000000000, 0.000000000000000000, 1.000000000000000000 ) ) ;
#8640=ORIENTED_EDGE ( 'NONE', *, *, #8754, .T. ) ;
#8642=VECTOR ( 'NONE', #6535, 1000.000000000000000 ) ;
#8648=ORIENTED_EDGE ( 'NONE', *, *, #2766, .T. ) ;
#8662=VECTOR ( 'NONE', #2011, 1000.000000000000000 ) ;
#8670=VERTEX_POINT ( 'NONE', #4460 ) ;
#8675=AXIS2_PLACEMENT_3D ( 'NONE', #630, #3736, #10152 ) ;
#8684=CARTESIAN_POINT ( 'NONE',  ( 0.000000000000000000, 216.0365690573663926, -15.00000000000000000 ) ) ;
#8687=CARTESIAN_POINT ( 'NONE',  ( 0.000000000000000000, 122.0000000000000000, 0.000000000000000000 ) ) ;
#8689=AXIS2_PLACEMENT_3D ( 'NONE', #4307, #5009, #2374 ) ;
#8697=CARTESIAN_POINT ( 'NONE',  ( 29.09218482426055985, 85.72793236853330257, 10.45696826948034008 ) ) ;
#8740=ORIENTED_EDGE ( 'NONE', *, *, #1177, .T. ) ;
#8743=CARTESIAN_POINT ( 'NONE',  ( 0.000000000000000000, 127.0000000000000000, 0.000000000000000000 ) ) ;
#8748=DIRECTION ( 'NONE',  ( -1.000000000000000000, 0.000000000000000000, 0.000000000000000000 ) ) ;
#8749=CARTESIAN_POINT ( 'NONE',  ( 27.96741528345890870, 86.27927944434865992, 11.41192941739706335 ) ) ;
#8754=EDGE_CURVE ( 'NONE', #12288, #4547, #8016, .T. ) ;
#8756=CARTESIAN_POINT ( 'NONE',  ( 2.694222958124177204E-15, 92.00000000000000000, 22.00000000000000355 ) ) ;
#8766=FACE_OUTER_BOUND ( 'NONE', #281, .T. ) ;
#8769=EDGE_CURVE ( 'NONE', #12062, #2119, #3028, .T. ) ;
#8787=LINE ( 'NONE', #7853, #2958 ) ;
#8804=ORIENTED_EDGE ( 'NONE', *, *, #8506, .T. ) ;
#8806=CARTESIAN_POINT ( 'NONE',  ( -13.00000000000000178, 170.0000000000000000, 7.483314773547879106 ) ) ;
#8821=CARTESIAN_POINT ( 'NONE',  ( -8.500000000000000000, 165.5000000000000000, 6.164414002968973350 ) ) ;
#8826=ADVANCED_FACE ( 'NONE', ( #7195 ), #4303, .T. ) ;
#8831=CYLINDRICAL_SURFACE ( 'NONE', #12009, 17.50000000000000000 ) ;
#8833=DIRECTION ( 'NONE',  ( 0.000000000000000000, 1.000000000000000000, 0.000000000000000000 ) ) ;
#8834=CARTESIAN_POINT ( 'NONE',  ( 27.94372984915585789, 86.14533704847936235, 11.47449158599552455 ) ) ;
#8845=ORIENTED_EDGE ( 'NONE', *, *, #4258, .F. ) ;
#8852=CARTESIAN_POINT ( 'NONE',  ( -34.73110591274434000, 77.00000000000000000, 8.660254037844445918 ) ) ;
#8871=DIRECTION ( 'NONE',  ( -0.000000000000000000, -1.000000000000000000, -0.000000000000000000 ) ) ;
#8873=VECTOR ( 'NONE', #8748, 1000.000000000000000 ) ;
#8897=CARTESIAN_POINT ( 'NONE',  ( 27.33018067101282966, 87.00000000000000000, 12.37179148263486539 ) ) ;
#8899=EDGE_CURVE ( 'NONE', #9385, #9969, #5320, .T. ) ;
#8931=VERTEX_POINT ( 'NONE', #4383 ) ;
#8939=CARTESIAN_POINT ( 'NONE',  ( 0.000000000000000000, 77.00000000000000000, 0.000000000000000000 ) ) ;
#8948=CARTESIAN_POINT ( 'NONE',  ( 27.53586651884002734, 87.45908356336218503, 11.91741659355933791 ) ) ;
#8953=VERTEX_POINT ( 'NONE', #12250 ) ;
#8956=CARTESIAN_POINT ( 'NONE',  ( -31.69148534550512863, 87.00819463772765516, -8.674447566738409776 ) ) ;
#8964=CARTESIAN_POINT ( 'NONE',  ( 28.72281323269012532, 87.00000000000000000, 8.660254037844435260 ) ) ;
#8988=ORIENTED_EDGE ( 'NONE', *, *, #10339, .F. ) ;
#9008=EDGE_LOOP ( 'NONE', ( #11105, #6939 ) ) ;
#9024=VERTEX_POINT ( 'NONE', #7325 ) ;
#9025=CARTESIAN_POINT ( 'NONE',  ( 31.23312648697674732, 87.04033007153441304, 8.730107770814976575 ) ) ;
#9026=CARTESIAN_POINT ( 'NONE',  ( 0.000000000000000000, 122.0000000000000000, 0.000000000000000000 ) ) ;
#9034=VERTEX_POINT ( 'NONE', #7387 ) ;
#9051=LINE ( 'NONE', #5457, #3201 ) ;
#9059=DIRECTION ( 'NONE',  ( 0.000000000000000000, 0.000000000000000000, 1.000000000000000000 ) ) ;
#9073=ADVANCED_FACE ( 'NONE', ( #3074 ), #4008, .F. ) ;
#9084=CARTESIAN_POINT ( 'NONE',  ( 0.000000000000000000, 127.0000000000000000, 0.000000000000000000 ) ) ;
#9092=CARTESIAN_POINT ( 'NONE',  ( -27.32050286291078933, 86.95679894682507438, -12.39317045950328477 ) ) ;
#9095=FACE_OUTER_BOUND ( 'NONE', #1947, .T. ) ;
#9113=ORIENTED_EDGE ( 'NONE', *, *, #8115, .T. ) ;
#9121=CARTESIAN_POINT ( 'NONE',  ( -27.31068353816013783, 86.91310272383458368, -12.41479448187959278 ) ) ;
#9122=CARTESIAN_POINT ( 'NONE',  ( 30.07733313487553772, 77.00000000000709122, -4.660254037819535178 ) ) ;
#9124=DIRECTION ( 'NONE',  ( -0.000000000000000000, 1.000000000000000000, -0.000000000000000000 ) ) ;
#9131=CARTESIAN_POINT ( 'NONE',  ( 27.67946139862178256, 88.39098822669899391, 11.04733141613932190 ) ) ;
#9133=CYLINDRICAL_SURFACE ( 'NONE', #5092, 22.00000000000000355 ) ;
#9139=CARTESIAN_POINT ( 'NONE',  ( -32.15778161310143446, 87.00000000000000000, -8.660254037844435260 ) ) ;
#9140=ORIENTED_EDGE ( 'NONE', *, *, #3609, .T. ) ;
#9149=ORIENTED_EDGE ( 'NONE', *, *, #5631, .F. ) ;
#9152=ORIENTED_EDGE ( 'NONE', *, *, #2974, .F. ) ;
#9170=DIRECTION ( 'NONE',  ( 0.000000000000000000, 1.000000000000000000, 0.000000000000000000 ) ) ;
#9177=ORIENTED_EDGE ( 'NONE', *, *, #8769, .F. ) ;
#9182=CARTESIAN_POINT ( 'NONE',  ( -30.12465603153679439, 85.44772375131798015, -9.971632707744779722 ) ) ;
#9185=CARTESIAN_POINT ( 'NONE',  ( -27.67946139862177546, 88.39098822669897970, -11.04733141613932901 ) ) ;
#9186=CARTESIAN_POINT ( 'NONE',  ( 1.836970198721029589E-15, 216.0365690573663926, 15.00000000000000000 ) ) ;
#9191=AXIS2_PLACEMENT_3D ( 'NONE', #8687, #3769, #1903 ) ;
#9196=FACE_OUTER_BOUND ( 'NONE', #11621, .T. ) ;
#9198=CARTESIAN_POINT ( 'NONE',  ( -32.15778161310143446, 87.00000000000000000, -8.660254037844435260 ) ) ;
#9213=DIRECTION ( 'NONE',  ( 0.000000000000000000, 1.000000000000000000, 0.000000000000000000 ) ) ;
#9214=CARTESIAN_POINT ( 'NONE',  ( -28.12254474901590484, 87.93978760833334718, -10.28801392380147206 ) ) ;
#9216=FACE_OUTER_BOUND ( 'NONE', #10664, .T. ) ;
#9221=EDGE_LOOP ( 'NONE', ( #12297, #954, #6988, #11939 ) ) ;
#9241=( LENGTH_UNIT ( ) NAMED_UNIT ( * ) SI_UNIT ( .MILLI., .METRE. ) );
#9243=DIRECTION ( 'NONE',  ( -0.000000000000000000, 1.000000000000000000, -0.000000000000000000 ) ) ;
#9249=CARTESIAN_POINT ( 'NONE',  ( -32.13993895771326947, 87.28197645339797361, -8.497454856569977011 ) ) ;
#9260=ORIENTED_EDGE ( 'NONE', *, *, #4016, .F. ) ;
#9262=CARTESIAN_POINT ( 'NONE',  ( -73.35315233757310693, 19.78571428571397917, -34.26986240689829089 ) ) ;
#9271=( BOUNDED_SURFACE ( )  B_SPLINE_SURFACE ( 3, 2, ( 
 ( #8258, #10187, #8192 ),
 ( #6274, #1661, #10121 ),
 ( #601, #8131, #4396 ),
 ( #9185, #5466, #9249 ) ),
 .UNSPECIFIED., .F., .F., .F. ) 
 B_SPLINE_SURFACE_WITH_KNOTS ( ( 4, 4 ),
 ( 3, 3 ),
 ( 0.08252307147639272034, 0.08572545668793904450 ),
 ( 0.000000000000000000, 1.000000000000000000 ),
 .UNSPECIFIED. ) 
 GEOMETRIC_REPRESENTATION_ITEM ( )  RATIONAL_B_SPLINE_SURFACE ( (
 ( 1.000000000000000000, 0.8237544710479142163, 1.000000000000000000),
 ( 1.000000000000000000, 0.8337078205039564205, 1.000000000000000000),
 ( 1.000000000000000000, 0.8426243553970728106, 1.000000000000000000),
 ( 1.000000000000000000, 0.8507194741069450394, 1.000000000000000000) ) ) 
 REPRESENTATION_ITEM ( '' )  SURFACE ( )  );
#9274=CARTESIAN_POINT ( 'NONE',  ( -8.500000000000000000, 165.5000000000000000, -7.483314773547880883 ) ) ;
#9283=DIRECTION ( 'NONE',  ( 0.000000000000000000, 0.000000000000000000, -1.000000000000000000 ) ) ;
#9285=PLANE ( 'NONE',  #5614 ) ;
#9290=DIRECTION ( 'NONE',  ( -0.000000000000000000, -0.4999999999999974465, 0.8660254037844401509 ) ) ;
#9300=EDGE_LOOP ( 'NONE', ( #1445, #2235, #9426, #10856 ) ) ;
#9302=( NAMED_UNIT ( * ) SI_UNIT ( $, .STERADIAN. ) SOLID_ANGLE_UNIT ( ) );
#9303=VECTOR ( 'NONE', #4300, 1000.000000000000000 ) ;
#9308=CARTESIAN_POINT ( 'NONE',  ( -30.14540500433760783, 76.99999999999997158, 4.927060346216586950 ) ) ;
#9311=CARTESIAN_POINT ( 'NONE',  ( -27.55156151032566214, 86.54395234961377525, -11.88489976664090442 ) ) ;
#9329=ORIENTED_EDGE ( 'NONE', *, *, #12329, .F. ) ;
#9330=EDGE_CURVE ( 'NONE', #8931, #7224, #7610, .T. ) ;
#9331=DIRECTION ( 'NONE',  ( 0.000000000000000000, 0.000000000000000000, 1.000000000000000000 ) ) ;
#9335=ORIENTED_EDGE ( 'NONE', *, *, #6315, .F. ) ;
#9336=EDGE_CURVE ( 'NONE', #1834, #7484, #10880, .T. ) ;
#9342=ORIENTED_EDGE ( 'NONE', *, *, #2759, .F. ) ;
#9345=AXIS2_PLACEMENT_3D ( 'NONE', #11047, #7248, #11111 ) ;
#9346=EDGE_CURVE ( 'NONE', #8931, #9024, #5869, .T. ) ;
#9353=DIRECTION ( 'NONE',  ( -0.000000000000000000, -1.000000000000000000, -0.000000000000000000 ) ) ;
#9368=SURFACE_SIDE_STYLE ('',( #3834 ) ) ;
#9370=ORIENTED_EDGE ( 'NONE', *, *, #10146, .F. ) ;
#9373=VECTOR ( 'NONE', #4993, 1000.000000000000000 ) ;
#9377=AXIS2_PLACEMENT_3D ( 'NONE', #1109, #3036, #6839 ) ;
#9383=DIRECTION ( 'NONE',  ( 0.000000000000000000, 0.000000000000000000, -1.000000000000000000 ) ) ;
#9385=VERTEX_POINT ( 'NONE', #7369 ) ;
#9402=CARTESIAN_POINT ( 'NONE',  ( 0.000000000000000000, 87.00000000000000000, 0.000000000000000000 ) ) ;
#9418=LINE ( 'NONE', #11435, #9561 ) ;
#9420=EDGE_CURVE ( 'NONE', #11122, #7224, #12097, .T. ) ;
#9426=ORIENTED_EDGE ( 'NONE', *, *, #8769, .T. ) ;
#9437=EDGE_CURVE ( 'NONE', #12186, #5470, #7984, .T. ) ;
#9445=LINE ( 'NONE', #1045, #3093 ) ;
#9459=FACE_OUTER_BOUND ( 'NONE', #2853, .T. ) ;
#9465=ADVANCED_FACE ( 'NONE', ( #4617 ), #7432, .F. ) ;
#9491=ADVANCED_FACE ( 'NONE', ( #6247 ), #7608, .F. ) ;
#9496=ORIENTED_EDGE ( 'NONE', *, *, #2787, .T. ) ;
#9506=CARTESIAN_POINT ( 'NONE',  ( 0.000000000000000000, 122.5000000000000000, 0.000000000000000000 ) ) ;
#9510=CARTESIAN_POINT ( 'NONE',  ( 0.000000000000000000, 170.0000000000000000, 0.000000000000000000 ) ) ;
#9511=ORIENTED_EDGE ( 'NONE', *, *, #1454, .T. ) ;
#9524=CARTESIAN_POINT ( 'NONE',  ( 73.35315233757310693, 79.55366347814538130, -0.2371791482635408899 ) ) ;
#9525=DIRECTION ( 'NONE',  ( -0.000000000000000000, -1.000000000000000000, -0.000000000000000000 ) ) ;
#9551=AXIS2_PLACEMENT_3D ( 'NONE', #11207, #7280, #6406 ) ;
#9561=VECTOR ( 'NONE', #4515, 1000.000000000000000 ) ;
#9562=CARTESIAN_POINT ( 'NONE',  ( 0.000000000000000000, 0.000000000000000000, 0.000000000000000000 ) ) ;
#9563=ADVANCED_FACE ( 'NONE', ( #10477 ), #948, .F. ) ;
#9569=CARTESIAN_POINT ( 'NONE',  ( 29.42287733398170602, 85.62135522733748871, 10.27237124600371487 ) ) ;
#9570=DIRECTION ( 'NONE',  ( 0.000000000000000000, -0.4999999999999976130, 0.8660254037844400399 ) ) ;
#9574=CARTESIAN_POINT ( 'NONE',  ( -32.18413411689675030, 86.41755723128771649, -8.996527527148016290 ) ) ;
#9593=EDGE_CURVE ( 'NONE', #10035, #9024, #7799, .T. ) ;
#9627=CARTESIAN_POINT ( 'NONE',  ( -29.63582346253862454, 77.00000000000000000, 4.660254037844413944 ) ) ;
#9644=CARTESIAN_POINT ( 'NONE',  ( 31.33267436902169933, 77.00000000000000000, -7.087639215986555108 ) ) ;
#9677=DIRECTION ( 'NONE',  ( 0.000000000000000000, -0.000000000000000000, 1.000000000000000000 ) ) ;
#9678=EDGE_LOOP ( 'NONE', ( #12215, #6036, #5215, #8458 ) ) ;
#9682=CARTESIAN_POINT ( 'NONE',  ( 30.00100000000000122, 77.00000000000000000, 8.660254037844445918 ) ) ;
#9700=CYLINDRICAL_SURFACE ( 'NONE', #3594, 10.49999999999999822 ) ;
#9723=CARTESIAN_POINT ( 'NONE',  ( 0.000000000000000000, 92.00000000000000000, -30.00000000000000000 ) ) ;
#9739=AXIS2_PLACEMENT_3D ( 'NONE', #2320, #11992, #1637 ) ;
#9746=( BOUNDED_CURVE ( )  B_SPLINE_CURVE ( 3, ( #534, #6148, #4330, #11950 ),
 .UNSPECIFIED., .F., .F. ) 
 B_SPLINE_CURVE_WITH_KNOTS ( ( 4, 4 ),
 ( 4.284962911267360397, 4.868362425771961099 ),
 .UNSPECIFIED. ) 
 CURVE ( )  GEOMETRIC_REPRESENTATION_ITEM ( )  RATIONAL_B_SPLINE_CURVE ( ( 1.000000000000000000, 0.9718376280744367435, 0.9718376280744367435, 1.000000000000000000 ) ) 
 REPRESENTATION_ITEM ( '' )  );
#9753=CARTESIAN_POINT ( 'NONE',  ( 30.50145854323926642, 85.38003226577610860, 9.854387615546505330 ) ) ;
#9769=CARTESIAN_POINT ( 'NONE',  ( 34.80930551369991122, 75.84619333735180646, -7.994103450571739877 ) ) ;
#9771=CARTESIAN_POINT ( 'NONE',  ( 27.57052686557079468, 86.63064495281062705, 11.84084938503489148 ) ) ;
#9782=CARTESIAN_POINT ( 'NONE',  ( 27.67899820261485999, 88.38261385519929547, 11.05501148229834030 ) ) ;
#9792=EDGE_LOOP ( 'NONE', ( #1548, #5961 ) ) ;
#9807=DIRECTION ( 'NONE',  ( 0.000000000000000000, 0.000000000000000000, 1.000000000000000000 ) ) ;
#9810=ORIENTED_EDGE ( 'NONE', *, *, #2019, .T. ) ;
#9814=CARTESIAN_POINT ( 'NONE',  ( 1.836970198721029589E-15, 127.0000000000000000, 15.00000000000000000 ) ) ;
#9815=DIRECTION ( 'NONE',  ( 0.000000000000000000, 0.000000000000000000, 1.000000000000000000 ) ) ;
#9817=CARTESIAN_POINT ( 'NONE',  ( 30.94187416189151918, 76.19472969970551901, -6.055023111780714729 ) ) ;
#9818=MECHANICAL_DESIGN_GEOMETRIC_PRESENTATION_REPRESENTATION('',(#1671),#11030);
#9822=ORIENTED_EDGE ( 'NONE', *, *, #9420, .F. ) ;
#9828=ORIENTED_EDGE ( 'NONE', *, *, #10354, .F. ) ;
#9830=CARTESIAN_POINT ( 'NONE',  ( 27.30089691780743877, 86.86968904112121947, 12.43627868308088935 ) ) ;
#9833=CARTESIAN_POINT ( 'NONE',  ( -27.88763417807736289, 88.17431669512683357, -10.69423021798056084 ) ) ;
#9838=ADVANCED_FACE ( 'NONE', ( #10945 ), #11203, .F. ) ;
#9841=CARTESIAN_POINT ( 'NONE',  ( 29.14112381217240255, 87.50172632198248834, 9.529269519012832035 ) ) ;
#9851=CARTESIAN_POINT ( 'NONE',  ( -29.75437749274565391, 83.76094350395922561, -7.050043618115805266 ) ) ;
#9853=VERTEX_POINT ( 'NONE', #1663 ) ;
#9854=DIRECTION ( 'NONE',  ( 0.000000000000000000, 0.000000000000000000, -1.000000000000000000 ) ) ;
#9867=FACE_OUTER_BOUND ( 'NONE', #2431, .T. ) ;
#9879=LINE ( 'NONE', #227, #10582 ) ;
#9885=DIRECTION ( 'NONE',  ( 0.000000000000000000, 0.000000000000000000, 1.000000000000000000 ) ) ;
#9889=B_SPLINE_CURVE_WITH_KNOTS ( 'NONE', 3,
 ( #11870, #4249, #1513, #1386 ),
 .UNSPECIFIED., .F., .F.,
 ( 4, 4 ),
 ( 0.000000000000000000, 0.002955678282115209009 ),
 .UNSPECIFIED. ) ;
#9893=CYLINDRICAL_SURFACE ( 'NONE', #11453, 15.00000000000000000 ) ;
#9898=CARTESIAN_POINT ( 'NONE',  ( -30.56632211525506904, 87.12700276260751764, -8.880229275382255594 ) ) ;
#9905=CARTESIAN_POINT ( 'NONE',  ( 31.69148534550512863, 87.00819463772768358, 8.674447566738409776 ) ) ;
#9916=EDGE_LOOP ( 'NONE', ( #10806, #5674, #1009, #10908 ) ) ;
#9917=CARTESIAN_POINT ( 'NONE',  ( -8.500000000000000000, 122.5000000000000000, 6.164414002968973350 ) ) ;
#9936=DIRECTION ( 'NONE',  ( 0.000000000000000000, 0.8660254037844407060, 0.4999999999999965583 ) ) ;
#9945=AXIS2_PLACEMENT_3D ( 'NONE', #7295, #2429, #432 ) ;
#9952=DIRECTION ( 'NONE',  ( 0.000000000000000000, 1.000000000000000000, 0.000000000000000000 ) ) ;
#9969=VERTEX_POINT ( 'NONE', #12265 ) ;
#9970=CARTESIAN_POINT ( 'NONE',  ( 2.081899558550500280E-15, 122.0000000000000000, -17.00000000000000000 ) ) ;
#9978=FACE_OUTER_BOUND ( 'NONE', #9221, .T. ) ;
#9981=CIRCLE ( 'NONE', #9377, 15.00000000000000000 ) ;
#10001=FACE_BOUND ( 'NONE', #5396, .T. ) ;
#10009=LINE ( 'NONE', #8076, #3273 ) ;
#10011=AXIS2_PLACEMENT_3D ( 'NONE', #4670, #4610, #7541 ) ;
#10018=CARTESIAN_POINT ( 'NONE',  ( 0.000000000000000000, 216.0365690573663926, 0.000000000000000000 ) ) ;
#10035=VERTEX_POINT ( 'NONE', #11639 ) ;
#10037=VECTOR ( 'NONE', #5299, 1000.000000000000000 ) ;
#10047=ORIENTED_EDGE ( 'NONE', *, *, #2787, .F. ) ;
#10048=CARTESIAN_POINT ( 'NONE',  ( 3.122849337825750222E-15, 87.00000000000000000, 25.50000000000000000 ) ) ;
#10059=CARTESIAN_POINT ( 'NONE',  ( 0.000000000000000000, 170.0000000000000000, 2.649999999999993694 ) ) ;
#10063=CIRCLE ( 'NONE', #7087, 2.649999999999987477 ) ;
#10064=CARTESIAN_POINT ( 'NONE',  ( -27.95322648060789206, 86.18856968700909249, -11.45194355884139448 ) ) ;
#10079=VERTEX_POINT ( 'NONE', #8749 ) ;
#10085=FACE_OUTER_BOUND ( 'NONE', #1058, .T. ) ;
#10089=CARTESIAN_POINT ( 'NONE',  ( -31.18707241436460365, 75.10640101998821194, 7.566984156997462740 ) ) ;
#10094=ORIENTED_EDGE ( 'NONE', *, *, #11885, .F. ) ;
#10100=AXIS2_PLACEMENT_3D ( 'NONE', #8216, #11100, #3438 ) ;
#10102=( GEOMETRIC_REPRESENTATION_CONTEXT ( 3 ) GLOBAL_UNCERTAINTY_ASSIGNED_CONTEXT ( ( #922 ) ) GLOBAL_UNIT_ASSIGNED_CONTEXT ( ( #12072, #5334, #12256 ) ) REPRESENTATION_CONTEXT ( 'NONE', 'WORKASPACE' ) );
#10105=LINE ( 'NONE', #2327, #1284 ) ;
#10115=ORIENTED_EDGE ( 'NONE', *, *, #4601, .F. ) ;
#10116=SURFACE_SIDE_STYLE ('',( #4575 ) ) ;
#10117=EDGE_CURVE ( 'NONE', #9034, #1793, #1414, .T. ) ;
#10120=CARTESIAN_POINT ( 'NONE',  ( 45.35898384862240107, 65.26794919243121740, -24.98076211353317078 ) ) ;
#10121=CARTESIAN_POINT ( 'NONE',  ( -32.12519652190516695, 85.41823950547528455, -9.573483885151777173 ) ) ;
#10134=ORIENTED_EDGE ( 'NONE', *, *, #7465, .T. ) ;
#10146=EDGE_CURVE ( 'NONE', #4534, #11714, #9051, .T. ) ;
#10150=EDGE_LOOP ( 'NONE', ( #1450, #11087, #9496, #7772 ) ) ;
#10152=DIRECTION ( 'NONE',  ( 5.551115123125782702E-15, -0.4999999999999976685, -0.8660254037844399289 ) ) ;
#10162=LINE ( 'NONE', #5196, #5182 ) ;
#10168=CARTESIAN_POINT ( 'NONE',  ( 0.000000000000000000, 87.00000000000000000, 0.000000000000000000 ) ) ;
#10169=VERTEX_POINT ( 'NONE', #11315 ) ;
#10176=TOROIDAL_SURFACE ( 'NONE', #6998, 24.99999999999999645, 5.000000000000000000 ) ;
#10187=CARTESIAN_POINT ( 'NONE',  ( -28.52887280570637074, 85.15789473684209554, -9.723794007404263695 ) ) ;
#10195=B_SPLINE_CURVE_WITH_KNOTS ( 'NONE', 3,
 ( #2223, #2401, #5966, #4277 ),
 .UNSPECIFIED., .F., .F.,
 ( 4, 4 ),
 ( 1.589900327696125378E-17, 0.001940928724149432009 ),
 .UNSPECIFIED. ) ;
#10199=CARTESIAN_POINT ( 'NONE',  ( 2.112515728529184067E-15, 122.5000000000000000, -17.00000000000000000 ) ) ;
#10210=ORIENTED_EDGE ( 'NONE', *, *, #7480, .F. ) ;
#10211=DIRECTION ( 'NONE',  ( 1.000000000000000000, -0.000000000000000000, 1.224646799147353207E-16 ) ) ;
#10216=FACE_OUTER_BOUND ( 'NONE', #8141, .T. ) ;
#10217=ORIENTED_EDGE ( 'NONE', *, *, #12180, .F. ) ;
#10223=ORIENTED_EDGE ( 'NONE', *, *, #8299, .T. ) ;
#10228=EDGE_CURVE ( 'NONE', #4839, #11632, #9418, .T. ) ;
#10229=VERTEX_POINT ( 'NONE', #5522 ) ;
#10232=CIRCLE ( 'NONE', #7054, 30.00000000000000000 ) ;
#10251=CARTESIAN_POINT ( 'NONE',  ( -27.57052686557075916, 86.63064495281066968, -11.84084938503495010 ) ) ;
#10259=AXIS2_PLACEMENT_3D ( 'NONE', #8743, #11509, #9677 ) ;
#10271=ADVANCED_FACE ( 'NONE', ( #2640 ), #6693, .T. ) ;
#10276=DIRECTION ( 'NONE',  ( 0.000000000000000000, 0.000000000000000000, -1.000000000000000000 ) ) ;
#10277=LINE ( 'NONE', #9274, #4435 ) ;
#10281=CARTESIAN_POINT ( 'NONE',  ( -28.72281323269012887, 87.00000000000000000, -8.660254037844435260 ) ) ;
#10289=EDGE_LOOP ( 'NONE', ( #11400, #6637, #7728, #2968, #6358, #757, #2208, #2948 ) ) ;
#10291=FACE_OUTER_BOUND ( 'NONE', #4029, .T. ) ;
#10293=CARTESIAN_POINT ( 'NONE',  ( 28.72281323269012532, 77.00000000000000000, -8.660254037844445918 ) ) ;
#10295=EDGE_LOOP ( 'NONE', ( #5627, #10223, #2051, #4481 ) ) ;
#10296=DIRECTION ( 'NONE',  ( 0.000000000000000000, 0.000000000000000000, 1.000000000000000000 ) ) ;
#10304=VERTEX_POINT ( 'NONE', #6514 ) ;
#10305=AXIS2_PLACEMENT_3D ( 'NONE', #2186, #10332, #10276 ) ;
#10320=CARTESIAN_POINT ( 'NONE',  ( 0.000000000000000000, 87.00000000000000000, 30.00000000000000000 ) ) ;
#10323=EDGE_LOOP ( 'NONE', ( #10115, #8740, #3867, #3800 ) ) ;
#10325=CARTESIAN_POINT ( 'NONE',  ( 27.30107202361637775, 86.87046582918780757, 12.43589427268144831 ) ) ;
#10330=DIRECTION ( 'NONE',  ( 0.000000000000000000, 0.000000000000000000, 1.000000000000000000 ) ) ;
#10332=DIRECTION ( 'NONE',  ( -0.000000000000000000, -1.000000000000000000, -0.000000000000000000 ) ) ;
#10339=EDGE_CURVE ( 'NONE', #9969, #10169, #6981, .T. ) ;
#10342=CARTESIAN_POINT ( 'NONE',  ( 0.000000000000000000, 127.0000000000000000, 0.000000000000000000 ) ) ;
#10354=EDGE_CURVE ( 'NONE', #9385, #9034, #7920, .T. ) ;
#10400=DIRECTION ( 'NONE',  ( 0.000000000000000000, -0.4999999999999974465, -0.8660254037844401509 ) ) ;
#10415=ORIENTED_EDGE ( 'NONE', *, *, #4877, .T. ) ;
#10428=CARTESIAN_POINT ( 'NONE',  ( 32.05000697088088657, 85.26794919243110371, 9.660254037844429931 ) ) ;
#10432=VECTOR ( 'NONE', #11428, 1000.000000000000000 ) ;
#10440=CARTESIAN_POINT ( 'NONE',  ( -33.79339916392899568, 75.30908861350523864, 7.588998470350058589 ) ) ;
#10451=EDGE_CURVE ( 'NONE', #4547, #12062, #1643, .T. ) ;
#10454=ORIENTED_EDGE ( 'NONE', *, *, #4341, .F. ) ;
#10463=( BOUNDED_SURFACE ( )  B_SPLINE_SURFACE ( 3, 2, ( 
 ( #5985, #9771, #114 ),
 ( #3989, #10776, #1246 ),
 ( #5054, #10593, #7663 ),
 ( #8834, #6045, #9830 ) ),
 .UNSPECIFIED., .F., .F., .F. ) 
 B_SPLINE_SURFACE_WITH_KNOTS ( ( 4, 4 ),
 ( 3, 3 ),
 ( 5.137468306293111020, 5.139829129961272614 ),
 ( 0.7666061298070568908, 1.000000000000000000 ),
 .UNSPECIFIED. ) 
 GEOMETRIC_REPRESENTATION_ITEM ( )  RATIONAL_B_SPLINE_SURFACE ( (
 ( 0.9369318869591325427, 0.9588653738936703252, 1.000000000000000000),
 ( 0.9369993130727707342, 0.9589093509185182551, 1.000000000000000000),
 ( 0.9370666800230418314, 0.9589532893555146043, 1.000000000000000000),
 ( 0.9371339877439250898, 0.9589971891615989286, 1.000000000000000000) ) ) 
 REPRESENTATION_ITEM ( '' )  SURFACE ( )  );
#10465=VECTOR ( 'NONE', #11283, 1000.000000000000000 ) ;
#10471=CARTESIAN_POINT ( 'NONE',  ( 30.83210227225915290, 77.00000000000000000, -6.426308247889123137 ) ) ;
#10477=FACE_OUTER_BOUND ( 'NONE', #11099, .T. ) ;
#10478=CARTESIAN_POINT ( 'NONE',  ( -28.72281323269012887, 87.00000000000000000, -8.660254037844435260 ) ) ;
#10485=ORIENTED_EDGE ( 'NONE', *, *, #6930, .F. ) ;
#10505=ADVANCED_FACE ( 'NONE', ( #9978 ), #635, .T. ) ;
#10511=CIRCLE ( 'NONE', #773, 17.00000000000000000 ) ;
#10520=CYLINDRICAL_SURFACE ( 'NONE', #10737, 2.649999999999993694 ) ;
#10523=ORIENTED_EDGE ( 'NONE', *, *, #9346, .F. ) ;
#10524=DIRECTION ( 'NONE',  ( 0.000000000000000000, 0.000000000000000000, 1.000000000000000000 ) ) ;
#10541=ADVANCED_FACE ( 'NONE', ( #7179 ), #10981, .F. ) ;
#10542=DIRECTION ( 'NONE',  ( -0.000000000000000000, -1.000000000000000000, -0.000000000000000000 ) ) ;
#10552=DIRECTION ( 'NONE',  ( -0.000000000000000000, -1.000000000000000000, -0.000000000000000000 ) ) ;
#10562=CARTESIAN_POINT ( 'NONE',  ( 0.000000000000000000, 122.0000000000000000, 0.000000000000000000 ) ) ;
#10563=CARTESIAN_POINT ( 'NONE',  ( -30.15809951803416666, 76.87504465863048608, 4.876683037773544172 ) ) ;
#10566=VECTOR ( 'NONE', #3195, 1000.000000000000000 ) ;
#10568=EDGE_LOOP ( 'NONE', ( #9260, #751, #1453, #5189 ) ) ;
#10574=DIRECTION ( 'NONE',  ( 0.000000000000000000, 0.8660254037844407060, -0.4999999999999965583 ) ) ;
#10582=VECTOR ( 'NONE', #1230, 1000.000000000000000 ) ;
#10587=VERTEX_POINT ( 'NONE', #7119 ) ;
#10588=CARTESIAN_POINT ( 'NONE',  ( 0.000000000000000000, 77.00000000000000000, 0.000000000000000000 ) ) ;
#10593=CARTESIAN_POINT ( 'NONE',  ( 27.55156151032568701, 86.54395234961377525, 11.88489976664085113 ) ) ;
#10605=ORIENTED_EDGE ( 'NONE', *, *, #4353, .F. ) ;
#10607=CARTESIAN_POINT ( 'NONE',  ( 27.33018067101282966, 87.00000000000000000, 12.37179148263486539 ) ) ;
#10611=ADVANCED_FACE ( 'NONE', ( #570 ), #420, .T. ) ;
#10615=CARTESIAN_POINT ( 'NONE',  ( 3.122849337825750222E-15, 77.00000000000000000, 25.50000000000000000 ) ) ;
#10621=CARTESIAN_POINT ( 'NONE',  ( 45.35898384862240107, 85.26794919243110371, 9.660254037844429931 ) ) ;
#10623=ORIENTED_EDGE ( 'NONE', *, *, #8044, .F. ) ;
#10626=CARTESIAN_POINT ( 'NONE',  ( -30.07733313487553772, 77.00000000000709122, 4.660254037819535178 ) ) ;
#10628=ORIENTED_EDGE ( 'NONE', *, *, #8044, .T. ) ;
#10629=COLOUR_RGB ( '', 0.72549020, 0.75294118, 0.79215686) ;
#10633=DIRECTION ( 'NONE',  ( -0.000000000000000000, -1.000000000000000000, -0.000000000000000000 ) ) ;
#10640=CARTESIAN_POINT ( 'NONE',  ( -45.35898384862240107, 85.26794919243110371, -9.660254037844419273 ) ) ;
#10646=CIRCLE ( 'NONE', #6067, 17.00000000000000000 ) ;
#10647=AXIS2_PLACEMENT_3D ( 'NONE', #6319, #10863, #5262 ) ;
#10648=ORIENTED_EDGE ( 'NONE', *, *, #6984, .T. ) ;
#10650=DIRECTION ( 'NONE',  ( -0.000000000000000000, -1.000000000000000000, -0.000000000000000000 ) ) ;
#10651=ORIENTED_EDGE ( 'NONE', *, *, #1886, .F. ) ;
#10664=EDGE_LOOP ( 'NONE', ( #9370, #10701, #3033, #12166 ) ) ;
#10672=EDGE_CURVE ( 'NONE', #7113, #10772, #8172, .T. ) ;
#10674=DIRECTION ( 'NONE',  ( 0.000000000000000000, -0.4999999999999974465, -0.8660254037844401509 ) ) ;
#10701=ORIENTED_EDGE ( 'NONE', *, *, #2085, .F. ) ;
#10708=CARTESIAN_POINT ( 'NONE',  ( -31.26438337082141672, 85.29075299833054657, -9.699751388268188279 ) ) ;
#10724=CYLINDRICAL_SURFACE ( 'NONE', #10305, 25.50000000000000000 ) ;
#10729=ORIENTED_EDGE ( 'NONE', *, *, #8491, .T. ) ;
#10732=CARTESIAN_POINT ( 'NONE',  ( -34.80930551369991122, 75.84619333735180646, 7.994103450571739877 ) ) ;
#10737=AXIS2_PLACEMENT_3D ( 'NONE', #9510, #7717, #1049 ) ;
#10739=ADVANCED_FACE ( 'NONE', ( #8290, #3564 ), #9285, .F. ) ;
#10744=CARTESIAN_POINT ( 'NONE',  ( 30.07733313487553772, 77.00000000000709122, -4.660254037819535178 ) ) ;
#10756=CIRCLE ( 'NONE', #4997, 10.49999999999999822 ) ;
#10766=EDGE_CURVE ( 'NONE', #1112, #4135, #3214, .T. ) ;
#10772=VERTEX_POINT ( 'NONE', #10478 ) ;
#10773=FACE_OUTER_BOUND ( 'NONE', #742, .T. ) ;
#10776=CARTESIAN_POINT ( 'NONE',  ( 27.56105762898382139, 86.58728811733513453, 11.86287969473300308 ) ) ;
#10778=CARTESIAN_POINT ( 'NONE',  ( -13.00000000000000178, 216.0365690573663926, 7.483314773547879106 ) ) ;
#10785=CARTESIAN_POINT ( 'NONE',  ( 28.78580657183880476, 87.64875042622801971, 9.783922737503322864 ) ) ;
#10787=ORIENTED_EDGE ( 'NONE', *, *, #1209, .T. ) ;
#10795=CARTESIAN_POINT ( 'NONE',  ( 0.000000000000000000, 92.00000000000000000, 0.000000000000000000 ) ) ;
#10796=TOROIDAL_SURFACE ( 'NONE', #9191, 17.00000000000000000, 0.5000000000000004441 ) ;
#10799=VERTEX_POINT ( 'NONE', #7792 ) ;
#10806=ORIENTED_EDGE ( 'NONE', *, *, #1760, .F. ) ;
#10811=EDGE_CURVE ( 'NONE', #12288, #7224, #5746, .T. ) ;
#10813=ORIENTED_EDGE ( 'NONE', *, *, #5520, .F. ) ;
#10816=CARTESIAN_POINT ( 'NONE',  ( 73.35315233757310693, 19.78571428571397917, 34.26986240689829089 ) ) ;
#10819=CARTESIAN_POINT ( 'NONE',  ( 30.25776724459628753, 76.75431408359612817, -5.085794527760020500 ) ) ;
#10822=AXIS2_PLACEMENT_3D ( 'NONE', #6456, #1593, #9059 ) ;
#10824=DIRECTION ( 'NONE',  ( -0.000000000000000000, -1.000000000000000000, -0.000000000000000000 ) ) ;
#10832=DIRECTION ( 'NONE',  ( 0.2207553928441711999, 0.8446598678744386968, -0.4876646020909775059 ) ) ;
#10837=CARTESIAN_POINT ( 'NONE',  ( 27.31079997599232456, 86.91362087007181003, 12.41453806599178478 ) ) ;
#10847=AXIS2_PLACEMENT_3D ( 'NONE', #7808, #3133, #10674 ) ;
#10856=ORIENTED_EDGE ( 'NONE', *, *, #8392, .T. ) ;
#10863=DIRECTION ( 'NONE',  ( 0.000000000000000000, 1.000000000000000000, 0.000000000000000000 ) ) ;
#10874=CARTESIAN_POINT ( 'NONE',  ( 0.000000000000000000, 87.00000000000000000, 0.000000000000000000 ) ) ;
#10880=CIRCLE ( 'NONE', #8689, 15.00000000000000000 ) ;
#10883=DIRECTION ( 'NONE',  ( 1.000000000000000000, -0.000000000000000000, 1.224646799147353207E-16 ) ) ;
#10884=CARTESIAN_POINT ( 'NONE',  ( 0.000000000000000000, 92.00000000000000000, 0.000000000000000000 ) ) ;
#10887=SHAPE_DEFINITION_REPRESENTATION ( #2790, #11842 ) ;
#10901=CARTESIAN_POINT ( 'NONE',  ( -29.92433840049366012, 87.25972750007186107, -9.110115264091719567 ) ) ;
#10906=CARTESIAN_POINT ( 'NONE',  ( 30.56632211525506548, 87.12700276260753185, 8.880229275382253817 ) ) ;
#10907=CARTESIAN_POINT ( 'NONE',  ( 0.000000000000000000, 165.5000000000000000, 0.000000000000000000 ) ) ;
#10908=ORIENTED_EDGE ( 'NONE', *, *, #5977, .F. ) ;
#10918=CARTESIAN_POINT ( 'NONE',  ( -30.00100000000000122, 75.26794919243111792, -7.660254037844449471 ) ) ;
#10921=EDGE_CURVE ( 'NONE', #5307, #4364, #11260, .T. ) ;
#10940=FACE_OUTER_BOUND ( 'NONE', #5428, .T. ) ;
#10941=CARTESIAN_POINT ( 'NONE',  ( 3.061616997868382648E-15, 87.00000000000000000, -24.99999999999999645 ) ) ;
#10944=CARTESIAN_POINT ( 'NONE',  ( 32.78711330112231792, 75.47285661897714704, -7.305343964218459440 ) ) ;
#10945=FACE_OUTER_BOUND ( 'NONE', #5770, .T. ) ;
#10970=LINE ( 'NONE', #6116, #9303 ) ;
#10974=CARTESIAN_POINT ( 'NONE',  ( 0.000000000000000000, 122.0000000000000000, 0.000000000000000000 ) ) ;
#10978=ORIENTED_EDGE ( 'NONE', *, *, #8899, .F. ) ;
#10981=PLANE ( 'NONE',  #6991 ) ;
#11002=CIRCLE ( 'NONE', #6035, 10.49999999999999822 ) ;
#11018=CIRCLE ( 'NONE', #5657, 0.5000000000000004441 ) ;
#11030=( GEOMETRIC_REPRESENTATION_CONTEXT ( 3 ) GLOBAL_UNCERTAINTY_ASSIGNED_CONTEXT ( ( #3405 ) ) GLOBAL_UNIT_ASSIGNED_CONTEXT ( ( #8494, #2765, #12316 ) ) REPRESENTATION_CONTEXT ( 'NONE', 'WORKASPACE' ) );
#11031=( BOUNDED_SURFACE ( )  B_SPLINE_SURFACE ( 3, 2, ( 
 ( #11981, #1685, #3553 ),
 ( #4423, #626, #12104 ),
 ( #7234, #1745, #688 ),
 ( #5365, #5430, #4545 ) ),
 .UNSPECIFIED., .F., .F., .F. ) 
 B_SPLINE_SURFACE_WITH_KNOTS ( ( 4, 4 ),
 ( 3, 3 ),
 ( 1.665911834627059607, 1.695449464845517618 ),
 ( 0.2468956587999593388, 1.000000000000000000 ),
 .UNSPECIFIED. ) 
 GEOMETRIC_REPRESENTATION_ITEM ( )  RATIONAL_B_SPLINE_SURFACE ( (
 ( 0.8800340755151767613, 0.7570513692546891882, 1.000000000000000000),
 ( 0.8788691223080344894, 0.7546921677749939272, 1.000000000000000000),
 ( 0.8776977286441711712, 0.7523199234237630817, 1.000000000000000000),
 ( 0.8765201392483088494, 0.7499351318045301973, 1.000000000000000000) ) ) 
 REPRESENTATION_ITEM ( '' )  SURFACE ( )  );
#11036=ORIENTED_EDGE ( 'NONE', *, *, #1177, .F. ) ;
#11038=FACE_OUTER_BOUND ( 'NONE', #3990, .T. ) ;
#11047=CARTESIAN_POINT ( 'NONE',  ( 0.000000000000000000, 127.0000000000000000, 0.000000000000000000 ) ) ;
#11054=CARTESIAN_POINT ( 'NONE',  ( 30.00100000000000122, 85.26794919243110371, -9.660254037844429931 ) ) ;
#11087=ORIENTED_EDGE ( 'NONE', *, *, #671, .T. ) ;
#11092=ORIENTED_EDGE ( 'NONE', *, *, #8754, .F. ) ;
#11099=EDGE_LOOP ( 'NONE', ( #993, #8648, #4051, #12255 ) ) ;
#11100=DIRECTION ( 'NONE',  ( 0.000000000000000000, 1.000000000000000000, 0.000000000000000000 ) ) ;
#11102=ORIENTED_EDGE ( 'NONE', *, *, #7229, .F. ) ;
#11105=ORIENTED_EDGE ( 'NONE', *, *, #11354, .F. ) ;
#11111=DIRECTION ( 'NONE',  ( 0.000000000000000000, 0.000000000000000000, -1.000000000000000000 ) ) ;
#11121=DIRECTION ( 'NONE',  ( 0.000000000000000000, -0.4999999999999976685, 0.8660254037844399289 ) ) ;
#11122=VERTEX_POINT ( 'NONE', #7532 ) ;
#11123=CARTESIAN_POINT ( 'NONE',  ( -28.72281323269012532, 77.00000000000000000, 8.660254037844445918 ) ) ;
#11147=LINE ( 'NONE', #7412, #8642 ) ;
#11152=CARTESIAN_POINT ( 'NONE',  ( 0.000000000000000000, 165.5000000000000000, 0.000000000000000000 ) ) ;
#11159=CIRCLE ( 'NONE', #7751, 40.00000000000000000 ) ;
#11177=AXIS2_PLACEMENT_3D ( 'NONE', #9402, #3741, #11419 ) ;
#11185=DIRECTION ( 'NONE',  ( 0.000000000000000000, 0.000000000000000000, 1.000000000000000000 ) ) ;
#11194=PRESENTATION_STYLE_ASSIGNMENT (( #1718 ) ) ;
#11201=CARTESIAN_POINT ( 'NONE',  ( -27.94372984915577618, 86.14533704847946183, -11.47449158599561692 ) ) ;
#11203=CYLINDRICAL_SURFACE ( 'NONE', #3220, 2.649999999999993694 ) ;
#11206=B_SPLINE_CURVE_WITH_KNOTS ( 'NONE', 3,
 ( #8285, #9214, #6494, #10281 ),
 .UNSPECIFIED., .F., .F.,
 ( 4, 4 ),
 ( 0.000000000000000000, 0.002955678282115210744 ),
 .UNSPECIFIED. ) ;
#11207=CARTESIAN_POINT ( 'NONE',  ( 45.35898384862240107, 67.00000000000008527, -25.98076211353315657 ) ) ;
#11217=AXIS2_PLACEMENT_3D ( 'NONE', #1486, #10832, #11784 ) ;
#11230=CARTESIAN_POINT ( 'NONE',  ( -29.94260118448502794, 78.56931597186009242, 5.428213010295147356 ) ) ;
#11249=DIRECTION ( 'NONE',  ( 0.000000000000000000, 1.000000000000000000, 0.000000000000000000 ) ) ;
#11255=B_SPLINE_CURVE_WITH_KNOTS ( 'NONE', 3,
 ( #9782, #3186, #7110, #6986, #10785, #9841, #2366, #4121, #1257, #5184, #10906, #7909, #9025, #9905, #11799, #2309 ),
 .UNSPECIFIED., .F., .F.,
 ( 4, 2, 2, 2, 2, 2, 2, 4 ),
 ( 0.000000000000000000, 0.001377885821436785046, 0.002066828732155181255, 0.002755771642873577464, 0.003444714553591973240, 0.004133657464310369449, 0.004822600375028765658, 0.005511543285747161867 ),
 .UNSPECIFIED. ) ;
#11260=B_SPLINE_CURVE_WITH_KNOTS ( 'NONE', 3,
 ( #620, #9833, #1557, #3367, #3238, #3177, #1368, #4171, #10901, #430, #9898, #11792, #2425, #8956, #7227, #9139 ),
 .UNSPECIFIED., .F., .F.,
 ( 4, 2, 2, 2, 2, 2, 2, 4 ),
 ( 0.000000000000000000, 0.001377885821436793719, 0.002066828732155186893, 0.002755771642873580500, 0.003444714553591973673, 0.004133657464310366847, 0.004822600375028760454, 0.005511543285747163602 ),
 .UNSPECIFIED. ) ;
#11282=LINE ( 'NONE', #9262, #2095 ) ;
#11283=DIRECTION ( 'NONE',  ( 0.000000000000000000, -0.8660254037844405950, -0.4999999999999965028 ) ) ;
#11289=CARTESIAN_POINT ( 'NONE',  ( 2.388061258337338939E-15, 127.0000000000000000, -17.00000000000000000 ) ) ;
#11294=DIRECTION ( 'NONE',  ( 0.000000000000000000, 0.000000000000000000, 1.000000000000000000 ) ) ;
#11298=CARTESIAN_POINT ( 'NONE',  ( -31.12930703771215235, 75.68563247576862807, 7.901403593909491541 ) ) ;
#11313=ADVANCED_FACE ( 'NONE', ( #7834 ), #10520, .F. ) ;
#11315=CARTESIAN_POINT ( 'NONE',  ( 0.000000000000000000, 127.0000000000000000, 17.00000000000000000 ) ) ;
#11321=PRESENTATION_STYLE_ASSIGNMENT (( #1900 ) ) ;
#11354=EDGE_CURVE ( 'NONE', #7018, #1569, #3770, .T. ) ;
#11358=DIRECTION ( 'NONE',  ( -0.2207553928441736979, 0.8446598678744383637, 0.4876646020909772838 ) ) ;
#11370=DIRECTION ( 'NONE',  ( 0.000000000000000000, 0.000000000000000000, -1.000000000000000000 ) ) ;
#11381=ADVANCED_FACE ( 'NONE', ( #1086 ), #5079, .T. ) ;
#11382=FILL_AREA_STYLE_COLOUR ( '', #10629 ) ;
#11389=CARTESIAN_POINT ( 'NONE',  ( -34.31149098582250190, 75.26794919243110371, 7.660254037844446806 ) ) ;
#11400=ORIENTED_EDGE ( 'NONE', *, *, #12329, .T. ) ;
#11403=VECTOR ( 'NONE', #1840, 1000.000000000000000 ) ;
#11407=AXIS2_PLACEMENT_3D ( 'NONE', #10907, #4424, #3494 ) ;
#11419=DIRECTION ( 'NONE',  ( 0.000000000000000000, 0.000000000000000000, 1.000000000000000000 ) ) ;
#11428=DIRECTION ( 'NONE',  ( -1.000000000000000000, 0.000000000000000000, 0.000000000000000000 ) ) ;
#11430=ORIENTED_EDGE ( 'NONE', *, *, #7229, .T. ) ;
#11435=CARTESIAN_POINT ( 'NONE',  ( -8.500000000000000000, 122.5000000000000000, -7.483314773547880883 ) ) ;
#11439=VERTEX_POINT ( 'NONE', #10615 ) ;
#11445=ORIENTED_EDGE ( 'NONE', *, *, #10228, .T. ) ;
#11446=FILL_AREA_STYLE ('',( #11382 ) ) ;
#11449=CARTESIAN_POINT ( 'NONE',  ( 30.00100000000000122, 85.26794919243110371, -9.660254037844429931 ) ) ;
#11453=AXIS2_PLACEMENT_3D ( 'NONE', #10018, #6917, #5116 ) ;
#11461=CYLINDRICAL_SURFACE ( 'NONE', #2655, 5.000000000000000000 ) ;
#11487=VERTEX_POINT ( 'NONE', #1208 ) ;
#11489=DIRECTION ( 'NONE',  ( 0.000000000000000000, -0.8660254037844400399, -0.4999999999999974465 ) ) ;
#11498=B_SPLINE_CURVE_WITH_KNOTS ( 'NONE', 3,
 ( #2531, #11949, #10708, #3530, #9182, #2339, #8253, #6147, #5919, #8189 ),
 .UNSPECIFIED., .F., .F.,
 ( 4, 2, 2, 2, 4 ),
 ( 2.797157557069881010E-17, 0.001173140257025626076, 0.002346280514051213555, 0.003519420771076801468, 0.004692561028102389814 ),
 .UNSPECIFIED. ) ;
#11501=CARTESIAN_POINT ( 'NONE',  ( 0.000000000000000000, 127.0000000000000000, -22.00000000000000355 ) ) ;
#11502=CARTESIAN_POINT ( 'NONE',  ( -27.69110892066586160, 86.46107124639166841, -11.72680205493506733 ) ) ;
#11505=EDGE_CURVE ( 'NONE', #2264, #6899, #9889, .T. ) ;
#11509=DIRECTION ( 'NONE',  ( 0.000000000000000000, 1.000000000000000000, 0.000000000000000000 ) ) ;
#11512=CARTESIAN_POINT ( 'NONE',  ( -13.00000000000000178, 127.0000000000000000, -7.483314773547880883 ) ) ;
#11514=DIRECTION ( 'NONE',  ( 0.000000000000000000, 1.000000000000000000, 0.000000000000000000 ) ) ;
#11515=EDGE_CURVE ( 'NONE', #8618, #12186, #10162, .T. ) ;
#11526=ORIENTED_EDGE ( 'NONE', *, *, #4405, .F. ) ;
#11529=ORIENTED_EDGE ( 'NONE', *, *, #5488, .F. ) ;
#11534=EDGE_CURVE ( 'NONE', #10229, #12186, #446, .T. ) ;
#11561=CARTESIAN_POINT ( 'NONE',  ( -27.30107202361637775, 86.87046582918780757, -12.43589427268144831 ) ) ;
#11572=CARTESIAN_POINT ( 'NONE',  ( 0.000000000000000000, 87.50000000000000000, 0.000000000000000000 ) ) ;
#11574=CARTESIAN_POINT ( 'NONE',  ( -34.84121487603211875, 75.26794919243111792, 7.660254037844449471 ) ) ;
#11578=B_SPLINE_CURVE_WITH_KNOTS ( 'NONE', 3,
 ( #6844, #9574, #2980, #4852 ),
 .UNSPECIFIED., .F., .F.,
 ( 4, 4 ),
 ( 0.000000000000000000, 0.002001274951694169586 ),
 .UNSPECIFIED. ) ;
#11582=EDGE_CURVE ( 'NONE', #4135, #3932, #3180, .T. ) ;
#11585=CARTESIAN_POINT ( 'NONE',  ( 69.85388127645428824, 17.99999999999971223, 31.17691453623957543 ) ) ;
#11597=ADVANCED_FACE ( 'NONE', ( #9095 ), #8104, .T. ) ;
#11603=CARTESIAN_POINT ( 'NONE',  ( 32.86043907464384972, 76.99999999999998579, -8.246007242324683517 ) ) ;
#11610=ORIENTED_EDGE ( 'NONE', *, *, #3073, .T. ) ;
#11621=EDGE_LOOP ( 'NONE', ( #4562, #6288, #12154, #7856 ) ) ;
#11632=VERTEX_POINT ( 'NONE', #9917 ) ;
#11639=CARTESIAN_POINT ( 'NONE',  ( -27.96741528345882344, 86.27927944434871677, -11.41192941739715927 ) ) ;
#11656=CIRCLE ( 'NONE', #6272, 17.50000000000000000 ) ;
#11663=FACE_OUTER_BOUND ( 'NONE', #3461, .T. ) ;
#11688=ORIENTED_EDGE ( 'NONE', *, *, #6169, .F. ) ;
#11690=EDGE_CURVE ( 'NONE', #7113, #7236, #807, .T. ) ;
#11698=DIRECTION ( 'NONE',  ( 0.000000000000000000, 0.000000000000000000, 1.000000000000000000 ) ) ;
#11713=CIRCLE ( 'NONE', #7720, 0.5000000000000004441 ) ;
#11714=VERTEX_POINT ( 'NONE', #2492 ) ;
#11718=LINE ( 'NONE', #1307, #4697 ) ;
#11724=PRODUCT_DEFINITION_FORMATION_WITH_SPECIFIED_SOURCE ( 'ANY', '', #207, .NOT_KNOWN. ) ;
#11734=CARTESIAN_POINT ( 'NONE',  ( 3.092233167847066435E-15, 87.50000000000000000, -24.99999999999999645 ) ) ;
#11757=AXIS2_PLACEMENT_3D ( 'NONE', #10795, #10552, #9854 ) ;
#11774=CARTESIAN_POINT ( 'NONE',  ( 0.000000000000000000, 122.5000000000000000, 17.00000000000000000 ) ) ;
#11784=DIRECTION ( 'NONE',  ( 0.000000000000000000, 0.4999999999999976685, 0.8660254037844399289 ) ) ;
#11792=CARTESIAN_POINT ( 'NONE',  ( -31.00813199677072163, 87.06416249055504863, -8.771386731425975469 ) ) ;
#11799=CARTESIAN_POINT ( 'NONE',  ( 31.92482683647866892, 87.00000000000011369, 8.660254037844589803 ) ) ;
#11800=PLANE ( 'NONE',  #11407 ) ;
#11802=DIRECTION ( 'NONE',  ( 0.000000000000000000, 0.000000000000000000, 1.000000000000000000 ) ) ;
#11815=LINE ( 'NONE', #3258, #1882 ) ;
#11820=AXIS2_PLACEMENT_3D ( 'NONE', #5431, #6546, #6489 ) ;
#11832=CARTESIAN_POINT ( 'NONE',  ( 32.32195836398363298, 75.59155356138302295, -7.099754829268524858 ) ) ;
#11842=SHAPE_REPRESENTATION ( 'Stainless Steel S-Blade Unit', ( #1612 ), #10102 ) ;
#11845=CARTESIAN_POINT ( 'NONE',  ( 0.000000000000000000, 127.0000000000000000, 0.000000000000000000 ) ) ;
#11850=ORIENTED_EDGE ( 'NONE', *, *, #10766, .T. ) ;
#11855=ORIENTED_EDGE ( 'NONE', *, *, #2888, .F. ) ;
#11859=CARTESIAN_POINT ( 'NONE',  ( 3.122849337825750222E-15, 92.00000000000000000, 25.50000000000000000 ) ) ;
#11869=VERTEX_POINT ( 'NONE', #11289 ) ;
#11870=CARTESIAN_POINT ( 'NONE',  ( 27.67899820261485999, 88.38261385519929547, 11.05501148229834030 ) ) ;
#11885=EDGE_CURVE ( 'NONE', #4534, #8555, #396, .T. ) ;
#11904=EDGE_LOOP ( 'NONE', ( #11850, #5632, #12102, #10210 ) ) ;
#11914=AXIS2_PLACEMENT_3D ( 'NONE', #2674, #754, #9331 ) ;
#11917=ORIENTED_EDGE ( 'NONE', *, *, #5597, .F. ) ;
#11939=ORIENTED_EDGE ( 'NONE', *, *, #1886, .T. ) ;
#11940=CARTESIAN_POINT ( 'NONE',  ( 0.000000000000000000, 170.0000000000000000, 0.000000000000000000 ) ) ;
#11949=CARTESIAN_POINT ( 'NONE',  ( -31.65330186654243505, 85.26794919243110371, -9.660254037844431707 ) ) ;
#11950=CARTESIAN_POINT ( 'NONE',  ( 29.63582346253862454, 77.00000000000000000, -4.660254037844413944 ) ) ;
#11966=CIRCLE ( 'NONE', #3596, 24.99999999999999645 ) ;
#11981=CARTESIAN_POINT ( 'NONE',  ( 30.08147999331295352, 76.80445198238156479, -4.520396356853239261 ) ) ;
#11983=EDGE_LOOP ( 'NONE', ( #4509, #7380, #4733, #1255, #7045, #3327, #7631 ) ) ;
#11992=DIRECTION ( 'NONE',  ( 1.000000000000000000, -0.000000000000000000, 1.224646799147353207E-16 ) ) ;
#12002=CARTESIAN_POINT ( 'NONE',  ( 0.000000000000000000, 87.50000000000000000, 24.99999999999999645 ) ) ;
#12009=AXIS2_PLACEMENT_3D ( 'NONE', #7660, #10650, #6728 ) ;
#12015=CARTESIAN_POINT ( 'NONE',  ( 34.31149098582250190, 75.26794919243110371, -7.660254037844446806 ) ) ;
#12016=ADVANCED_FACE ( 'NONE', ( #8766 ), #3106, .T. ) ;
#12024=AXIS2_PLACEMENT_3D ( 'NONE', #10941, #10883, #283 ) ;
#12038=AXIS2_PLACEMENT_3D ( 'NONE', #11152, #12279, #1795 ) ;
#12039=EDGE_LOOP ( 'NONE', ( #10523, #3030, #998 ) ) ;
#12043=CARTESIAN_POINT ( 'NONE',  ( 30.00100000000000122, 77.00000000000000000, 8.660254037844445918 ) ) ;
#12048=VECTOR ( 'NONE', #10542, 1000.000000000000000 ) ;
#12049=CARTESIAN_POINT ( 'NONE',  ( -27.31079997599232456, 86.91362087007181003, -12.41453806599178655 ) ) ;
#12062=VERTEX_POINT ( 'NONE', #2114 ) ;
#12072=( LENGTH_UNIT ( ) NAMED_UNIT ( * ) SI_UNIT ( .MILLI., .METRE. ) );
#12074=ADVANCED_FACE ( 'NONE', ( #5915 ), #9700, .F. ) ;
#12086=ORIENTED_EDGE ( 'NONE', *, *, #7597, .F. ) ;
#12092=DIRECTION ( 'NONE',  ( -0.000000000000000000, -1.000000000000000000, -0.000000000000000000 ) ) ;
#12093=DIRECTION ( 'NONE',  ( 1.000000000000000000, 0.000000000000000000, 0.000000000000000000 ) ) ;
#12097=CIRCLE ( 'NONE', #4522, 30.00000000000000000 ) ;
#12102=ORIENTED_EDGE ( 'NONE', *, *, #2279, .T. ) ;
#12104=CARTESIAN_POINT ( 'NONE',  ( 34.80906958247980754, 75.85155757747834571, -7.997200496052795593 ) ) ;
#12109=CARTESIAN_POINT ( 'NONE',  ( -30.03968734988933420, 77.39454232463201322, 4.824121477407818048 ) ) ;
#12125=FACE_OUTER_BOUND ( 'NONE', #230, .T. ) ;
#12138=CARTESIAN_POINT ( 'NONE',  ( -32.61619934561887391, 76.99999999999998579, 8.120688671832020589 ) ) ;
#12141=DIRECTION ( 'NONE',  ( 0.000000000000000000, 0.000000000000000000, 1.000000000000000000 ) ) ;
#12146=FACE_OUTER_BOUND ( 'NONE', #10295, .T. ) ;
#12152=CARTESIAN_POINT ( 'NONE',  ( 0.000000000000000000, 122.5000000000000000, 0.000000000000000000 ) ) ;
#12154=ORIENTED_EDGE ( 'NONE', *, *, #5488, .T. ) ;
#12165=CARTESIAN_POINT ( 'NONE',  ( 0.000000000000000000, 165.5000000000000000, 0.000000000000000000 ) ) ;
#12166=ORIENTED_EDGE ( 'NONE', *, *, #2975, .F. ) ;
#12180=EDGE_CURVE ( 'NONE', #5955, #9853, #10756, .T. ) ;
#12186=VERTEX_POINT ( 'NONE', #1482 ) ;
#12201=CARTESIAN_POINT ( 'NONE',  ( -30.23169114332096896, 76.99999999999998579, 5.192055827170280580 ) ) ;
#12212=CARTESIAN_POINT ( 'NONE',  ( 29.63582346253862454, 77.00000000000000000, -4.660254037844413944 ) ) ;
#12215=ORIENTED_EDGE ( 'NONE', *, *, #1836, .F. ) ;
#12225=DIRECTION ( 'NONE',  ( 0.000000000000000000, 0.000000000000000000, 1.000000000000000000 ) ) ;
#12234=DIRECTION ( 'NONE',  ( 0.000000000000000000, 0.8660254037844407060, -0.4999999999999965028 ) ) ;
#12240=DIRECTION ( 'NONE',  ( -0.000000000000000000, -0.4999999999999974465, 0.8660254037844401509 ) ) ;
#12250=CARTESIAN_POINT ( 'NONE',  ( -13.00000000000000178, 170.0000000000000000, -7.483314773547880883 ) ) ;
#12251=CARTESIAN_POINT ( 'NONE',  ( -8.500000000000000000, 216.0365690573663926, -7.483314773547880883 ) ) ;
#12255=ORIENTED_EDGE ( 'NONE', *, *, #3334, .F. ) ;
#12256=( NAMED_UNIT ( * ) SI_UNIT ( $, .STERADIAN. ) SOLID_ANGLE_UNIT ( ) );
#12258=DIRECTION ( 'NONE',  ( -0.000000000000000000, -1.000000000000000000, -0.000000000000000000 ) ) ;
#12265=CARTESIAN_POINT ( 'NONE',  ( 2.694222958124177204E-15, 122.0000000000000000, 22.00000000000000355 ) ) ;
#12279=DIRECTION ( 'NONE',  ( 0.000000000000000000, 1.000000000000000000, 0.000000000000000000 ) ) ;
#12288=VERTEX_POINT ( 'NONE', #4532 ) ;
#12291=ORIENTED_EDGE ( 'NONE', *, *, #10228, .F. ) ;
#12293=CARTESIAN_POINT ( 'NONE',  ( 0.000000000000000000, 216.0365690573663926, -10.49999999999999822 ) ) ;
#12297=ORIENTED_EDGE ( 'NONE', *, *, #4955, .F. ) ;
#12313=VECTOR ( 'NONE', #498, 1000.000000000000000 ) ;
#12316=( NAMED_UNIT ( * ) SI_UNIT ( $, .STERADIAN. ) SOLID_ANGLE_UNIT ( ) );
#12318=ORIENTED_EDGE ( 'NONE', *, *, #11515, .T. ) ;
#12329=EDGE_CURVE ( 'NONE', #2134, #4117, #6971, .T. ) ;
#12333=CARTESIAN_POINT ( 'NONE',  ( 28.20745110743105499, 86.12135132227002998, 11.13838988601293778 ) ) ;
#12344=ADVANCED_FACE ( 'NONE', ( #12146 ), #670, .F. ) ;
#12353=CARTESIAN_POINT ( 'NONE',  ( -45.35898384862240107, 67.00000000000008527, 25.98076211353315657 ) ) ;
ENDSEC;
END-ISO-10303-21;
